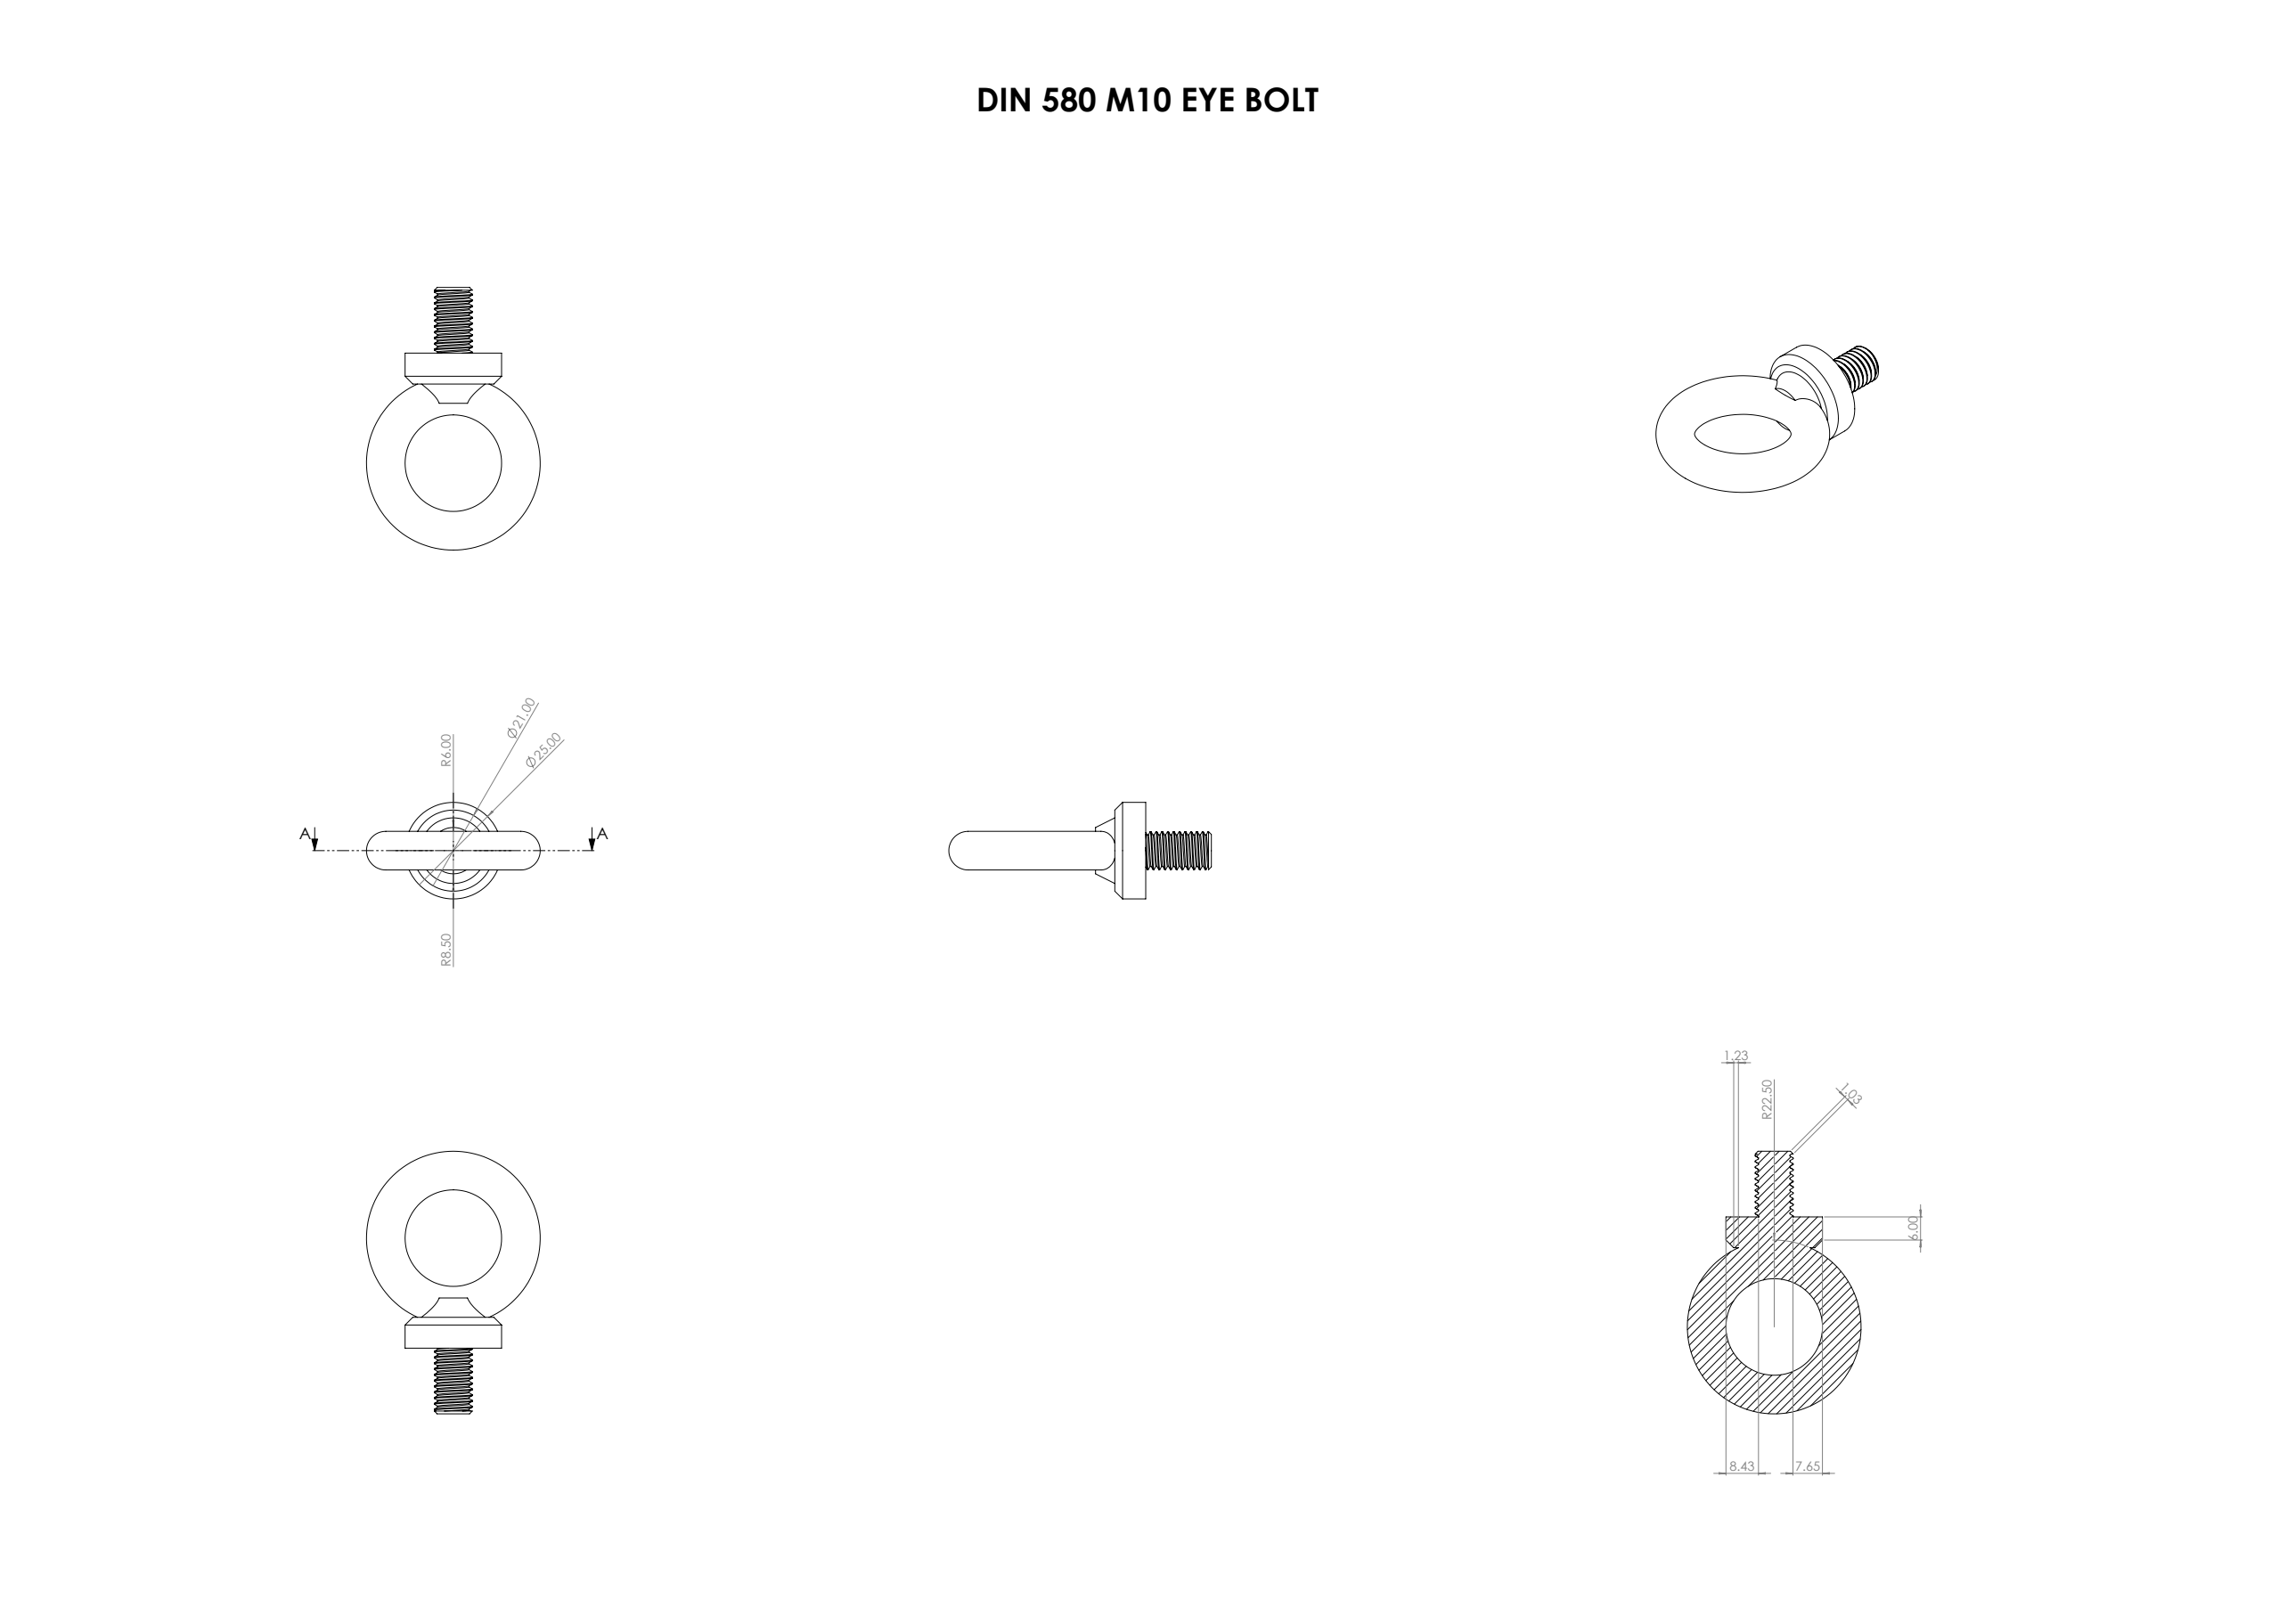
ISO-10303-21;
HEADER;
/* Generated by software containing ST-Developer
 * from STEP Tools, Inc. (www.steptools.com) 
 */

FILE_DESCRIPTION(
/* description */ (''),
/* implementation_level */ '2;1');

FILE_NAME(
/* name */ '15_DIN_580_M10_Eye_Bolt.step',
/* time_stamp */ '2026-10-20T10:03:03-07:00',
/* author */ (''),
/* organization */ (''),
/* preprocessor_version */ 'ST-DEVELOPER v20.2',
/* originating_system */ 'Autodesk Translation Framework v15.15.0.0',
/* authorisation */ '');

FILE_SCHEMA (('AUTOMOTIVE_DESIGN { 1 0 10303 214 3 1 1 }'));
ENDSEC;

DATA;
#10=MECHANICAL_DESIGN_GEOMETRIC_PRESENTATION_REPRESENTATION('',(#537),#71492);
#380=TOROIDAL_SURFACE('',#30209,1.75,0.5);
#394=SHAPE_REPRESENTATION_RELATIONSHIP('SRR','None',#71615,#413);
#413=ADVANCED_BREP_SHAPE_REPRESENTATION('',(#432),#71485);
#432=MANIFOLD_SOLID_BREP('Eye bolt',#28471);
#537=STYLED_ITEM('',(#71894),#432);
#909=B_SPLINE_CURVE_WITH_KNOTS('',3,(#56996,#56997,#56998,#56999,#57000,
#57001,#57002,#57003,#57004,#57005),.UNSPECIFIED.,.F.,.F.,(4,3,3,4),(-4.09323272002469,
-3.95713141738306,-2.9678485630373,-2.06652207565085),.UNSPECIFIED.);
#910=B_SPLINE_CURVE_WITH_KNOTS('',3,(#57008,#57009,#57010,#57011,#57012,
#57013,#57014,#57015,#57016,#57017),.UNSPECIFIED.,.F.,.F.,(4,3,3,4),(0.,
0.494641427172876,0.989282854345763,1.11488200921591),.UNSPECIFIED.);
#911=B_SPLINE_CURVE_WITH_KNOTS('',3,(#57022,#57023,#57024,#57025,#57026,
#57027,#57028,#57029,#57030,#57031,#57032,#57033,#57034,#57035,#57036,#57037,
#57038,#57039,#57040,#57041,#57042,#57043),.UNSPECIFIED.,.F.,.F.,(4,3,3,
3,3,3,3,4),(-10.3764180272043,-9.89282854345765,-8.90354568911189,-7.91426283476612,
-6.92497998042036,-5.93569712607459,-4.94641427172883,-4.09323272002469),
 .UNSPECIFIED.);
#912=B_SPLINE_CURVE_WITH_KNOTS('',3,(#57044,#57045,#57046,#57047,#57048,
#57049,#57050,#57051,#57052,#57053,#57054,#57055,#57056,#57057,#57058,#57059,
#57060,#57061,#57062,#57063,#57064,#57065),.UNSPECIFIED.,.F.,.F.,(4,3,3,
3,3,3,3,4),(1.11488200921591,1.97856570869153,2.9678485630373,3.95713141738306,
4.94641427172883,5.93569712607459,6.92497998042036,7.39806731639549),
 .UNSPECIFIED.);
#913=B_SPLINE_CURVE_WITH_KNOTS('',3,(#57070,#57071,#57072,#57073,#57074,
#57075,#57076,#57077,#57078,#57079,#57080,#57081,#57082,#57083,#57084,#57085,
#57086,#57087,#57088,#57089,#57090,#57091),.UNSPECIFIED.,.F.,.F.,(4,3,3,
3,3,3,3,4),(-16.6596033343839,-15.8285256695322,-14.8392428151865,-13.8499599608407,
-12.860677106495,-11.8713942521492,-10.8821113978034,-10.3764180272043),
 .UNSPECIFIED.);
#914=B_SPLINE_CURVE_WITH_KNOTS('',3,(#57092,#57093,#57094,#57095,#57096,
#57097,#57098,#57099,#57100,#57101,#57102,#57103,#57104,#57105,#57106,#57107,
#57108,#57109,#57110,#57111,#57112,#57113),.UNSPECIFIED.,.F.,.F.,(4,3,3,
3,3,3,3,4),(7.39806731639549,7.91426283476612,8.90354568911189,9.89282854345766,
10.8821113978034,11.8713942521492,12.860677106495,13.6812526235751),
 .UNSPECIFIED.);
#915=B_SPLINE_CURVE_WITH_KNOTS('',3,(#57118,#57119,#57120,#57121,#57122,
#57123,#57124,#57125,#57126,#57127,#57128,#57129,#57130,#57131,#57132,#57133,
#57134,#57135,#57136,#57137,#57138,#57139,#57140,#57141,#57142),
 .UNSPECIFIED.,.F.,.F.,(4,3,3,3,3,3,3,3,4),(-22.9427886415635,-22.7535056499526,
-21.7642227956068,-20.7749399412611,-19.7856570869153,-18.7963742325695,
-17.8070913782238,-16.817808523878,-16.6596033343839),.UNSPECIFIED.);
#916=B_SPLINE_CURVE_WITH_KNOTS('',3,(#57143,#57144,#57145,#57146,#57147,
#57148,#57149,#57150,#57151,#57152,#57153,#57154,#57155,#57156,#57157,#57158,
#57159,#57160,#57161,#57162,#57163,#57164,#57165,#57166,#57167),
 .UNSPECIFIED.,.F.,.F.,(4,3,3,3,3,3,3,3,4),(13.6812526235751,13.8499599608407,
14.8392428151865,15.8285256695323,16.817808523878,17.8070913782238,18.7963742325695,
19.7856570869153,19.9644379307547),.UNSPECIFIED.);
#917=B_SPLINE_CURVE_WITH_KNOTS('',3,(#57172,#57173,#57174,#57175,#57176,
#57177,#57178,#57179,#57180,#57181,#57182,#57183,#57184,#57185,#57186,#57187,
#57188,#57189,#57190,#57191,#57192,#57193),.UNSPECIFIED.,.F.,.F.,(4,3,3,
3,3,3,3,4),(-29.225973948743,-28.6892027760272,-27.6999199216814,-26.7106370673357,
-25.7213542129899,-24.7320713586441,-23.7427885042984,-22.9427886415635),
 .UNSPECIFIED.);
#918=B_SPLINE_CURVE_WITH_KNOTS('',3,(#57194,#57195,#57196,#57197,#57198,
#57199,#57200,#57201,#57202,#57203,#57204,#57205,#57206,#57207,#57208,#57209,
#57210,#57211,#57212,#57213,#57214,#57215),.UNSPECIFIED.,.F.,.F.,(4,3,3,
3,3,3,3,4),(19.9644379307547,20.7749399412611,21.7642227956068,22.7535056499526,
23.7427885042984,24.7320713586441,25.7213542129899,26.2476232379343),
 .UNSPECIFIED.);
#919=B_SPLINE_CURVE_WITH_KNOTS('',3,(#57220,#57221,#57222,#57223,#57224,
#57225,#57226,#57227,#57228,#57229,#57230,#57231,#57232,#57233,#57234,#57235,
#57236,#57237,#57238,#57239,#57240,#57241),.UNSPECIFIED.,.F.,.F.,(4,3,3,
3,3,3,3,4),(-35.5091592559226,-34.6248999021018,-33.635617047756,-32.6463341934103,
-31.6570513390645,-30.6677684847187,-29.678485630373,-29.225973948743),
 .UNSPECIFIED.);
#920=B_SPLINE_CURVE_WITH_KNOTS('',3,(#57242,#57243,#57244,#57245,#57246,
#57247,#57248,#57249,#57250,#57251,#57252,#57253,#57254,#57255,#57256,#57257,
#57258,#57259,#57260,#57261,#57262,#57263),.UNSPECIFIED.,.F.,.F.,(4,3,3,
3,3,3,3,4),(26.2476232379343,26.7106370673357,27.6999199216814,28.6892027760272,
29.678485630373,30.6677684847187,31.6570513390645,32.5308085451138),
 .UNSPECIFIED.);
#921=B_SPLINE_CURVE_WITH_KNOTS('',3,(#57268,#57269,#57270,#57271,#57272,
#57273,#57274,#57275,#57276,#57277,#57278,#57279,#57280,#57281,#57282,#57283,
#57284,#57285,#57286,#57287,#57288,#57289,#57290,#57291,#57292),
 .UNSPECIFIED.,.F.,.F.,(4,3,3,3,3,3,3,3,4),(-41.7923445631022,-41.5498798825222,
-40.5605970281764,-39.5713141738306,-38.5820313194849,-37.5927484651391,
-36.6034656107933,-35.6141827564476,-35.5091592559226),.UNSPECIFIED.);
#922=B_SPLINE_CURVE_WITH_KNOTS('',3,(#57293,#57294,#57295,#57296,#57297,
#57298,#57299,#57300,#57301,#57302,#57303,#57304,#57305,#57306,#57307,#57308,
#57309,#57310,#57311,#57312,#57313,#57314,#57315,#57316,#57317),
 .UNSPECIFIED.,.F.,.F.,(4,3,3,3,3,3,3,3,4),(32.5308085451138,32.6463341934103,
33.635617047756,34.6248999021018,35.6141827564476,36.6034656107933,37.5927484651391,
38.5820313194849,38.8139938522934),.UNSPECIFIED.);
#923=B_SPLINE_CURVE_WITH_KNOTS('',3,(#57322,#57323,#57324,#57325,#57326,
#57327,#57328,#57329,#57330,#57331,#57332,#57333,#57334,#57335,#57336,#57337,
#57338,#57339,#57340,#57341,#57342,#57343),.UNSPECIFIED.,.F.,.F.,(4,3,3,
3,3,3,3,4),(-48.0755298702818,-47.4855770085967,-46.496294154251,-45.5070112999052,
-44.5177284455594,-43.5284455912137,-42.5391627368679,-41.7923445631022),
 .UNSPECIFIED.);
#924=B_SPLINE_CURVE_WITH_KNOTS('',3,(#57344,#57345,#57346,#57347,#57348,
#57349,#57350,#57351,#57352,#57353,#57354,#57355,#57356,#57357,#57358,#57359,
#57360,#57361,#57362,#57363,#57364,#57365),.UNSPECIFIED.,.F.,.F.,(4,3,3,
3,3,3,3,4),(38.8139938522934,39.5713141738306,40.5605970281764,41.5498798825221,
42.5391627368679,43.5284455912137,44.5177284455594,45.097179159473),
 .UNSPECIFIED.);
#925=B_SPLINE_CURVE_WITH_KNOTS('',3,(#57370,#57371,#57372,#57373,#57374,
#57375,#57376,#57377,#57378,#57379,#57380,#57381,#57382,#57383,#57384,#57385,
#57386,#57387,#57388,#57389,#57390,#57391),.UNSPECIFIED.,.F.,.F.,(4,3,3,
3,3,3,3,4),(-54.3587151774614,-53.4212741346713,-52.4319912803256,-51.4427084259798,
-50.453425571634,-49.4641427172883,-48.4748598629425,-48.0755298702818),
 .UNSPECIFIED.);
#926=B_SPLINE_CURVE_WITH_KNOTS('',3,(#57392,#57393,#57394,#57395,#57396,
#57397,#57398,#57399,#57400,#57401,#57402,#57403,#57404,#57405,#57406,#57407,
#57408,#57409,#57410,#57411,#57412,#57413),.UNSPECIFIED.,.F.,.F.,(4,3,3,
3,3,3,3,4),(45.097179159473,45.5070112999052,46.496294154251,47.4855770085967,
48.4748598629425,49.4641427172883,50.4534255716341,51.3803644666526),
 .UNSPECIFIED.);
#927=B_SPLINE_CURVE_WITH_KNOTS('',3,(#57418,#57419,#57420,#57421,#57422,
#57423,#57424,#57425,#57426,#57427,#57428,#57429,#57430,#57431,#57432,#57433,
#57434,#57435,#57436,#57437,#57438,#57439,#57440,#57441,#57442),
 .UNSPECIFIED.,.F.,.F.,(4,3,3,3,3,3,3,3,4),(-60.641900484641,-60.3462541150917,
-59.3569712607459,-58.3676884064002,-57.3784055520544,-56.3891226977086,
-55.3998398433629,-54.4105569890171,-54.3587151774614),.UNSPECIFIED.);
#928=B_SPLINE_CURVE_WITH_KNOTS('',3,(#57443,#57444,#57445,#57446,#57447,
#57448,#57449,#57450,#57451,#57452,#57453,#57454,#57455,#57456,#57457,#57458,
#57459,#57460,#57461,#57462,#57463,#57464,#57465,#57466,#57467),
 .UNSPECIFIED.,.F.,.F.,(4,3,3,3,3,3,3,3,4),(51.3803644666526,51.4427084259798,
52.4319912803256,53.4212741346713,54.4105569890171,55.3998398433629,56.3891226977086,
57.3784055520544,57.6635497738322),.UNSPECIFIED.);
#929=B_SPLINE_CURVE_WITH_KNOTS('',3,(#57472,#57473,#57474,#57475,#57476,
#57477,#57478,#57479,#57480,#57481,#57482,#57483,#57484,#57485,#57486,#57487,
#57488,#57489,#57490,#57491,#57492,#57493),.UNSPECIFIED.,.F.,.F.,(4,3,3,
3,3,3,3,4),(-66.9250857918206,-66.2819512411663,-65.2926683868205,-64.3033855324747,
-63.314102678129,-62.3248198237832,-61.3355369694375,-60.641900484641),
 .UNSPECIFIED.);
#930=B_SPLINE_CURVE_WITH_KNOTS('',3,(#57494,#57495,#57496,#57497,#57498,
#57499,#57500,#57501,#57502,#57503,#57504,#57505,#57506,#57507,#57508,#57509,
#57510,#57511,#57512,#57513,#57514,#57515),.UNSPECIFIED.,.F.,.F.,(4,3,3,
3,3,3,3,4),(57.6635497738322,58.3676884064002,59.3569712607459,60.3462541150917,
61.3355369694375,62.3248198237832,63.314102678129,63.9467350810118),
 .UNSPECIFIED.);
#931=B_SPLINE_CURVE_WITH_KNOTS('',3,(#57521,#57522,#57523,#57524,#57525),
 .UNSPECIFIED.,.F.,.F.,(4,1,4),(78.5398163397448,78.8859646434363,79.7872911308227),
 .UNSPECIFIED.);
#932=B_SPLINE_CURVE_WITH_KNOTS('',3,(#57528,#57529,#57530,#57531),
 .UNSPECIFIED.,.F.,.F.,(4,4),(78.5398163397448,78.5489786101027),
 .UNSPECIFIED.);
#933=B_SPLINE_CURVE_WITH_KNOTS('',3,(#57536,#57537,#57538,#57539,#57540,
#57541,#57542,#57543,#57544,#57545),.UNSPECIFIED.,.F.,.F.,(4,1,1,1,1,1,
1,4),(72.2566310325653,72.9502675173617,73.9395503717074,74.9288332260532,
75.918116080399,76.9073989347447,77.8966817890905,78.5398163397448),
 .UNSPECIFIED.);
#934=B_SPLINE_CURVE_WITH_KNOTS('',3,(#57546,#57547,#57548,#57549,#57550,
#57551,#57552,#57553,#57554,#57555,#57556),.UNSPECIFIED.,.F.,.F.,(4,1,1,
1,1,1,1,1,4),(72.2566310325652,72.6132814840281,73.6025643383739,74.5918471927197,
75.5811300470654,76.5704129014112,77.5596957557569,78.0543371829298,78.5398163397448),
 .UNSPECIFIED.);
#935=B_SPLINE_CURVE_WITH_KNOTS('',3,(#57561,#57562,#57563,#57564,#57565,
#57566,#57567,#57568,#57569,#57570,#57571),.UNSPECIFIED.,.F.,.F.,(4,1,1,
1,1,1,1,1,4),(65.9734457253856,66.0252875369413,67.0145703912871,68.0038532456329,
68.9931360999786,69.9824189543244,70.9717018086701,71.9609846630159,72.2566310325653),
 .UNSPECIFIED.);
#936=B_SPLINE_CURVE_WITH_KNOTS('',3,(#57572,#57573,#57574,#57575,#57576,
#57577,#57578,#57579,#57580,#57581),.UNSPECIFIED.,.F.,.F.,(4,1,1,1,1,1,
1,4),(65.9734457253856,66.6775843579535,67.6668672122993,68.6561500666451,
69.6454329209908,70.6347157753366,71.6239986296824,72.2566310325652),
 .UNSPECIFIED.);
#937=B_SPLINE_CURVE_WITH_KNOTS('',3,(#57586,#57587,#57588,#57589,#57590,
#57591,#57592,#57593,#57594,#57595),.UNSPECIFIED.,.F.,.F.,(4,1,1,1,1,1,
1,4),(59.6902604182061,60.0895904108667,61.0788732652125,62.0681561195583,
63.057438973904,64.0467218282498,65.0360046825956,65.9734457253856),
 .UNSPECIFIED.);
#938=B_SPLINE_CURVE_WITH_KNOTS('',3,(#57596,#57597,#57598,#57599,#57600,
#57601,#57602,#57603,#57604,#57605,#57606),.UNSPECIFIED.,.F.,.F.,(4,1,1,
1,1,1,1,1,4),(59.6902604182061,59.7526043775332,60.7418872318789,61.7311700862247,
62.7204529405705,63.7097357949162,64.699018649262,65.6883015036078,65.9734457253856),
 .UNSPECIFIED.);
#939=B_SPLINE_CURVE_WITH_KNOTS('',3,(#57611,#57612,#57613,#57614,#57615,
#57616,#57617,#57618,#57619,#57620),.UNSPECIFIED.,.F.,.F.,(4,1,1,1,1,1,
1,4),(53.4070751110265,54.1538932847921,55.1431761391379,56.1324589934837,
57.1217418478294,58.1110247021752,59.100307556521,59.6902604182061),
 .UNSPECIFIED.);
#940=B_SPLINE_CURVE_WITH_KNOTS('',3,(#57621,#57622,#57623,#57624,#57625,
#57626,#57627,#57628,#57629,#57630),.UNSPECIFIED.,.F.,.F.,(4,1,1,1,1,1,
1,4),(53.4070751110265,53.8169072514586,54.8061901058043,55.7954729601501,
56.7847558144959,57.7740386688416,58.7633215231874,59.6902604182061),
 .UNSPECIFIED.);
#941=B_SPLINE_CURVE_WITH_KNOTS('',3,(#57635,#57636,#57637,#57638,#57639,
#57640,#57641,#57642,#57643,#57644,#57645),.UNSPECIFIED.,.F.,.F.,(4,1,1,
1,1,1,1,1,4),(47.1238898038469,47.2289133043718,48.2181961587175,49.2074790130633,
50.1967618674091,51.1860447217548,52.1753275761006,53.1646104304464,53.4070751110265),
 .UNSPECIFIED.);
#942=B_SPLINE_CURVE_WITH_KNOTS('',3,(#57646,#57647,#57648,#57649,#57650,
#57651,#57652,#57653,#57654,#57655),.UNSPECIFIED.,.F.,.F.,(4,1,1,1,1,1,
1,4),(47.1238898038469,47.881210125384,48.8704929797298,49.8597758340755,
50.8490586884213,51.8383415427671,52.8276243971128,53.4070751110265),
 .UNSPECIFIED.);
#943=B_SPLINE_CURVE_WITH_KNOTS('',3,(#57660,#57661,#57662,#57663,#57664,
#57665,#57666,#57667,#57668,#57669),.UNSPECIFIED.,.F.,.F.,(4,1,1,1,1,1,
1,4),(40.8407044966673,41.2932161782972,42.2824990326429,43.2717818869887,
44.2610647413345,45.2503475956803,46.239630450026,47.1238898038469),
 .UNSPECIFIED.);
#944=B_SPLINE_CURVE_WITH_KNOTS('',3,(#57670,#57671,#57672,#57673,#57674,
#57675,#57676,#57677,#57678,#57679,#57680),.UNSPECIFIED.,.F.,.F.,(4,1,1,
1,1,1,1,1,4),(40.8407044966673,40.9562301449636,41.9455129993094,42.9347958536552,
43.9240787080009,44.9133615623467,45.9026444166925,46.8919272710382,47.1238898038469),
 .UNSPECIFIED.);
#945=B_SPLINE_CURVE_WITH_KNOTS('',3,(#57685,#57686,#57687,#57688,#57689,
#57690,#57691,#57692,#57693,#57694),.UNSPECIFIED.,.F.,.F.,(4,1,1,1,1,1,
1,4),(34.5575191894877,35.3575190522226,36.3468019065684,37.3360847609141,
38.3253676152599,39.3146504696057,40.3039333239514,40.8407044966673),
 .UNSPECIFIED.);
#946=B_SPLINE_CURVE_WITH_KNOTS('',3,(#57695,#57696,#57697,#57698,#57699,
#57700,#57701,#57702,#57703,#57704),.UNSPECIFIED.,.F.,.F.,(4,1,1,1,1,1,
1,4),(34.5575191894877,35.020533018889,36.0098158732348,36.9990987275806,
37.9883815819263,38.9776644362721,39.9669472906179,40.8407044966673),
 .UNSPECIFIED.);
#947=B_SPLINE_CURVE_WITH_KNOTS('',3,(#57709,#57710,#57711,#57712,#57713,
#57714,#57715,#57716,#57717,#57718,#57719),.UNSPECIFIED.,.F.,.F.,(4,1,1,
1,1,1,1,1,4),(28.2743338823081,28.4325390718022,29.421821926148,30.4111047804938,
31.4003876348395,32.3896704891853,33.3789533435311,34.3682361978768,34.5575191894877),
 .UNSPECIFIED.);
#948=B_SPLINE_CURVE_WITH_KNOTS('',3,(#57720,#57721,#57722,#57723,#57724,
#57725,#57726,#57727,#57728,#57729),.UNSPECIFIED.,.F.,.F.,(4,1,1,1,1,1,
1,4),(28.2743338823081,29.0848358928144,30.0741187471602,31.063401601506,
32.0526844558517,33.0419673101975,34.0312501645433,34.5575191894877),
 .UNSPECIFIED.);
#949=B_SPLINE_CURVE_WITH_KNOTS('',3,(#57734,#57735,#57736,#57737,#57738,
#57739,#57740,#57741,#57742,#57743),.UNSPECIFIED.,.F.,.F.,(4,1,1,1,1,1,
1,4),(21.9911485751285,22.4968419457276,23.4861248000734,24.4754076544192,
25.4646905087649,26.4539733631107,27.4432562174565,28.2743338823081),
 .UNSPECIFIED.);
#950=B_SPLINE_CURVE_WITH_KNOTS('',3,(#57744,#57745,#57746,#57747,#57748,
#57749,#57750,#57751,#57752,#57753,#57754),.UNSPECIFIED.,.F.,.F.,(4,1,1,
1,1,1,1,1,4),(21.9911485751285,22.1598559123941,23.1491387667399,24.1384216210856,
25.1277044754314,26.1169873297771,27.1062701841229,28.0955530384687,28.2743338823081),
 .UNSPECIFIED.);
#951=B_SPLINE_CURVE_WITH_KNOTS('',3,(#57759,#57760,#57761,#57762,#57763,
#57764,#57765,#57766,#57767,#57768),.UNSPECIFIED.,.F.,.F.,(4,1,1,1,1,1,
1,4),(15.7079632679489,16.561144819653,17.5504276739988,18.5397105283446,
19.5289933826903,20.5182762370361,21.5075590913819,21.9911485751285),
 .UNSPECIFIED.);
#952=B_SPLINE_CURVE_WITH_KNOTS('',3,(#57769,#57770,#57771,#57772,#57773,
#57774,#57775,#57776,#57777,#57778),.UNSPECIFIED.,.F.,.F.,(4,1,1,1,1,1,
1,4),(15.7079632679489,16.2241587863195,17.2134416406653,18.202724495011,
19.1920073493568,20.1812902037026,21.1705730580483,21.9911485751285),
 .UNSPECIFIED.);
#953=B_SPLINE_CURVE_WITH_KNOTS('',3,(#57784,#57785,#57786,#57787,#57788,
#57789),.UNSPECIFIED.,.F.,.F.,(4,2,4),(-0.342456092017903,-0.262804961413355,
0.),.UNSPECIFIED.);
#954=B_SPLINE_CURVE_WITH_KNOTS('',3,(#57791,#57792,#57793,#57794,#57795,
#57796,#57797,#57798,#57799,#57800,#57801,#57802),.UNSPECIFIED.,.F.,.F.,
(4,2,2,2,2,4),(0.,0.178010957135692,0.381093675614414,0.596885981784515,
0.750004601526435,0.833159445966906),.UNSPECIFIED.);
#955=B_SPLINE_CURVE_WITH_KNOTS('',3,(#57804,#57805,#57806,#57807,#57808,
#57809,#57810,#57811,#57812,#57813,#57814,#57815,#57816,#57817),
 .UNSPECIFIED.,.F.,.F.,(4,2,2,2,2,2,4),(2.8879030854515,2.90631755511173,
3.01588868292827,3.10104216567944,3.18619564843061,3.29576677624714,3.31418124590738),
 .UNSPECIFIED.);
#956=B_SPLINE_CURVE_WITH_KNOTS('',3,(#57819,#57820,#57821,#57822,#57823,
#57824,#57825,#57826,#57827,#57828,#57829,#57830),.UNSPECIFIED.,.F.,.F.,
(4,2,2,2,2,4),(0.,0.182810359067708,0.452655692105918,0.783610652837132,
0.960006030065839,1.14418486243573),.UNSPECIFIED.);
#957=B_SPLINE_CURVE_WITH_KNOTS('',3,(#57832,#57833,#57834,#57835,#57836,
#57837),.UNSPECIFIED.,.F.,.F.,(4,2,4),(3.5322737051841,3.79507866659746,
3.87472979720201),.UNSPECIFIED.);
#958=B_SPLINE_CURVE_WITH_KNOTS('',3,(#57841,#57842,#57843,#57844,#57845,
#57846),.UNSPECIFIED.,.F.,.F.,(4,2,4),(3.1898176131662,3.26946874377075,
3.5322737051841),.UNSPECIFIED.);
#959=B_SPLINE_CURVE_WITH_KNOTS('',3,(#57848,#57849,#57850,#57851,#57852,
#57853,#57854,#57855,#57856,#57857,#57858,#57859),.UNSPECIFIED.,.F.,.F.,
(4,2,2,2,2,4),(0.,0.178010957135693,0.381093675614418,0.59688598178454,
0.750004601526475,0.833159445966973),.UNSPECIFIED.);
#960=B_SPLINE_CURVE_WITH_KNOTS('',3,(#57861,#57862,#57863,#57864,#57865,
#57866,#57867,#57868,#57869,#57870,#57871,#57872,#57873,#57874),
 .UNSPECIFIED.,.F.,.F.,(4,2,2,2,2,2,4),(0.820541641665208,0.838956111325442,
0.948527239141976,1.03368072189315,1.11883420464432,1.22840533246085,1.24681980212109),
 .UNSPECIFIED.);
#961=B_SPLINE_CURVE_WITH_KNOTS('',3,(#57876,#57877,#57878,#57879,#57880,
#57881,#57882,#57883,#57884,#57885,#57886,#57887),.UNSPECIFIED.,.F.,.F.,
(4,2,2,2,2,4),(0.,0.182810359067185,0.452655692103104,0.783610652831579,
0.960006030058821,1.14418486242717),.UNSPECIFIED.);
#962=B_SPLINE_CURVE_WITH_KNOTS('',3,(#57888,#57889,#57890,#57891,#57892,
#57893),.UNSPECIFIED.,.F.,.F.,(4,2,4),(0.,0.262804961413355,0.342456092017903),
 .UNSPECIFIED.);
#963=B_SPLINE_CURVE_WITH_KNOTS('',3,(#57909,#57910,#57911,#57912,#57913,
#57914,#57915,#57916,#57917,#57918,#57919,#57920,#57921,#57922,#57923,#57924,
#57925,#57926,#57927,#57928,#57929,#57930,#57931,#57932,#57933,#57934,#57935,
#57936,#57937,#57938,#57939,#57940,#57941,#57942,#57943,#57944,#57945,#57946,
#57947,#57948,#57949,#57950,#57951,#57952,#57953,#57954,#57955,#57956,#57957,
#57958,#57959,#57960,#57961,#57962,#57963,#57964,#57965,#57966,#57967,#57968,
#57969,#57970,#57971,#57972,#57973,#57974,#57975),.UNSPECIFIED.,.F.,.F.,
(4,3,3,3,3,3,3,3,3,3,3,3,3,3,3,3,3,3,3,3,3,3,4),(-0.93774096308181,-0.870261948404392,
-0.832251019814623,-0.812039353702878,-0.742348954142412,-0.729339847034109,
-0.705081468871194,-0.634283519265674,-0.572488451018333,-0.549579435213131,
-0.530963570226855,-0.510693382770993,-0.438960472290944,-0.388997500739232,
-0.372134856040166,-0.354858390446,-0.276993114348998,-0.218594157276247,
-0.196204166307054,-0.17703031168743,-0.099567067450566,-0.043397286057993,
0.),.UNSPECIFIED.);
#964=B_SPLINE_CURVE_WITH_KNOTS('',3,(#57977,#57978,#57979,#57980,#57981,
#57982,#57983,#57984,#57985,#57986,#57987,#57988,#57989,#57990,#57991,#57992,
#57993,#57994,#57995,#57996,#57997,#57998,#57999,#58000,#58001,#58002,#58003,
#58004,#58005,#58006,#58007,#58008,#58009,#58010,#58011,#58012,#58013,#58014,
#58015,#58016,#58017,#58018,#58019,#58020,#58021,#58022,#58023,#58024,#58025,
#58026,#58027,#58028,#58029,#58030,#58031,#58032,#58033,#58034,#58035,#58036,
#58037,#58038,#58039,#58040,#58041,#58042,#58043),.UNSPECIFIED.,.F.,.F.,
(4,3,3,3,3,3,3,3,3,3,3,3,3,3,3,3,3,3,3,3,3,3,4),(-0.933975894023158,-0.856824867797122,
-0.821914501343845,-0.791558113020374,-0.71597790947688,-0.694994410329363,
-0.668582197141203,-0.594616471062628,-0.530120471538128,-0.507052841767612,
-0.490181983238915,-0.465624472013627,-0.393047138731511,-0.348092731553511,
-0.32871533726739,-0.312541480427752,-0.242076479471633,-0.190609197809111,
-0.162579557995071,-0.14514061306184,-0.078314656879451,-0.0362073528215457,
0.),.UNSPECIFIED.);
#965=B_SPLINE_CURVE_WITH_KNOTS('',3,(#58356,#58357,#58358,#58359,#58360,
#58361,#58362,#58363,#58364),.UNSPECIFIED.,.F.,.F.,(4,1,1,1,1,1,4),(11.6147305479242,
12.1093719750971,12.60401340227,13.5932962566158,14.5825791109615,15.5718619653073,
15.7079632679489),.UNSPECIFIED.);
#966=B_SPLINE_CURVE_WITH_KNOTS('',3,(#58365,#58366,#58367,#58368,#58369,
#58370,#58371,#58372,#58373,#58374,#58375,#58376,#58377,#58378,#58379,#58380,
#58381,#58382,#58383,#58384,#58385,#58386,#58387,#58388,#58389,#58390,#58391,
#58392,#58393,#58394,#58395,#58396,#58397,#58398,#58399,#58400,#58401,#58402,
#58403,#58404,#58405,#58406,#58407,#58408,#58409,#58410,#58411,#58412,#58413,
#58414,#58415,#58416,#58417,#58418,#58419,#58420,#58421,#58422,#58423,#58424,
#58425,#58426,#58427,#58428,#58429,#58430,#58431),.UNSPECIFIED.,.F.,.F.,
(4,3,3,3,3,3,3,3,3,3,3,3,3,3,3,3,3,3,3,3,3,3,4),(-0.933975894023119,-0.890767895830556,
-0.832649055223636,-0.807165334613026,-0.784870232004528,-0.708420338291616,
-0.684040660118115,-0.663611018024939,-0.589324938941615,-0.542495792243922,
-0.504321658003645,-0.487154884783798,-0.425817170975192,-0.367338377334077,
-0.338840187897342,-0.316929096908672,-0.246728742864094,-0.207915887991521,
-0.16973711093609,-0.149619355722235,-0.0812991141899627,-0.0146711098764389,
0.),.UNSPECIFIED.);
#967=B_SPLINE_CURVE_WITH_KNOTS('',3,(#58432,#58433,#58434,#58435,#58436,
#58437,#58438,#58439,#58440,#58441,#58442,#58443,#58444,#58445,#58446,#58447),
 .UNSPECIFIED.,.F.,.F.,(4,3,3,3,3,4),(-70.2390826585493,-69.7444412313765,
-69.2497998042036,-68.2605169498578,-67.2712340955121,-66.9250857918206),
 .UNSPECIFIED.);
#968=B_SPLINE_CURVE_WITH_KNOTS('',3,(#58450,#58451,#58452,#58453,#58454,
#58455,#58456,#58457,#58458),.UNSPECIFIED.,.F.,.F.,(4,1,1,1,1,1,4),(10.3764180272042,
11.2777445145907,12.2670273689364,13.2563102232822,14.245593077628,15.2348759319737,
15.7079632679489),.UNSPECIFIED.);
#969=B_SPLINE_CURVE_WITH_KNOTS('',3,(#58764,#58765,#58766,#58767,#58768,
#58769,#58770,#58771,#58772,#58773,#58774,#58775,#58776,#58777,#58778,#58779),
 .UNSPECIFIED.,.F.,.F.,(4,3,3,3,3,4),(63.9467350810118,64.3033855324747,
65.2926683868205,66.2819512411663,67.2712340955121,68.1725605828985),
 .UNSPECIFIED.);
#970=B_SPLINE_CURVE_WITH_KNOTS('',3,(#58780,#58781,#58782,#58783,#58784,
#58785,#58786,#58787,#58788,#58789,#58790,#58791,#58792,#58793,#58794,#58795,
#58796,#58797,#58798,#58799,#58800,#58801,#58802,#58803,#58804,#58805,#58806,
#58807,#58808,#58809,#58810,#58811,#58812,#58813,#58814,#58815,#58816,#58817,
#58818,#58819,#58820,#58821,#58822,#58823,#58824,#58825,#58826,#58827,#58828,
#58829,#58830,#58831,#58832,#58833,#58834,#58835,#58836,#58837,#58838,#58839,
#58840,#58841,#58842,#58843),.UNSPECIFIED.,.F.,.F.,(4,3,3,3,3,3,3,3,3,3,
3,3,3,3,3,3,3,3,3,3,3,4),(-0.937740963081774,-0.901429380350922,-0.842615939984195,
-0.815134419970695,-0.763821611298058,-0.734138838750838,-0.715144480290609,
-0.643654231153057,-0.571972635037333,-0.551702893088566,-0.534998195849319,
-0.470725533976372,-0.413107434862205,-0.384514347555702,-0.359013510944126,
-0.284551929400665,-0.240253137519706,-0.200676800014282,-0.176385565585146,
-0.0995853117506865,-0.0229257113100043,0.),.UNSPECIFIED.);
#1462=B_SPLINE_SURFACE_WITH_KNOTS('',3,3,((#58051,#58052,#58053,#58054,
#58055,#58056,#58057,#58058,#58059,#58060,#58061,#58062,#58063,#58064,#58065,
#58066,#58067,#58068,#58069,#58070,#58071,#58072,#58073,#58074,#58075,#58076,
#58077,#58078,#58079,#58080,#58081,#58082,#58083,#58084,#58085,#58086,#58087,
#58088,#58089,#58090,#58091,#58092,#58093,#58094,#58095,#58096,#58097,#58098,
#58099,#58100,#58101,#58102,#58103,#58104,#58105,#58106,#58107,#58108,#58109,
#58110,#58111,#58112,#58113,#58114,#58115,#58116,#58117,#58118,#58119,#58120,
#58121,#58122,#58123,#58124,#58125,#58126),(#58127,#58128,#58129,#58130,
#58131,#58132,#58133,#58134,#58135,#58136,#58137,#58138,#58139,#58140,#58141,
#58142,#58143,#58144,#58145,#58146,#58147,#58148,#58149,#58150,#58151,#58152,
#58153,#58154,#58155,#58156,#58157,#58158,#58159,#58160,#58161,#58162,#58163,
#58164,#58165,#58166,#58167,#58168,#58169,#58170,#58171,#58172,#58173,#58174,
#58175,#58176,#58177,#58178,#58179,#58180,#58181,#58182,#58183,#58184,#58185,
#58186,#58187,#58188,#58189,#58190,#58191,#58192,#58193,#58194,#58195,#58196,
#58197,#58198,#58199,#58200,#58201,#58202),(#58203,#58204,#58205,#58206,
#58207,#58208,#58209,#58210,#58211,#58212,#58213,#58214,#58215,#58216,#58217,
#58218,#58219,#58220,#58221,#58222,#58223,#58224,#58225,#58226,#58227,#58228,
#58229,#58230,#58231,#58232,#58233,#58234,#58235,#58236,#58237,#58238,#58239,
#58240,#58241,#58242,#58243,#58244,#58245,#58246,#58247,#58248,#58249,#58250,
#58251,#58252,#58253,#58254,#58255,#58256,#58257,#58258,#58259,#58260,#58261,
#58262,#58263,#58264,#58265,#58266,#58267,#58268,#58269,#58270,#58271,#58272,
#58273,#58274,#58275,#58276,#58277,#58278),(#58279,#58280,#58281,#58282,
#58283,#58284,#58285,#58286,#58287,#58288,#58289,#58290,#58291,#58292,#58293,
#58294,#58295,#58296,#58297,#58298,#58299,#58300,#58301,#58302,#58303,#58304,
#58305,#58306,#58307,#58308,#58309,#58310,#58311,#58312,#58313,#58314,#58315,
#58316,#58317,#58318,#58319,#58320,#58321,#58322,#58323,#58324,#58325,#58326,
#58327,#58328,#58329,#58330,#58331,#58332,#58333,#58334,#58335,#58336,#58337,
#58338,#58339,#58340,#58341,#58342,#58343,#58344,#58345,#58346,#58347,#58348,
#58349,#58350,#58351,#58352,#58353,#58354)),.UNSPECIFIED.,.F.,.F.,.F.,(4,
4),(4,1,1,1,1,1,1,1,1,1,1,1,1,1,1,1,1,1,1,1,1,1,1,1,1,1,1,1,1,1,1,1,1,1,
1,1,1,1,1,1,1,1,1,1,1,1,1,1,1,1,1,1,1,1,1,1,1,1,1,1,1,1,1,1,1,1,1,1,1,1,
1,1,1,4),(0.,0.0986691610045069),(11.6147305479242,12.1093719750971,12.60401340227,
13.5932962566158,14.5825791109615,15.5718619653073,16.561144819653,17.5504276739988,
18.5397105283446,19.5289933826903,20.5182762370361,21.5075590913819,22.4968419457276,
23.4861248000734,24.4754076544192,25.4646905087649,26.4539733631107,27.4432562174565,
28.4325390718022,29.421821926148,30.4111047804938,31.4003876348395,32.3896704891853,
33.3789533435311,34.3682361978768,35.3575190522226,36.3468019065684,37.3360847609141,
38.3253676152599,39.3146504696057,40.3039333239514,41.2932161782972,42.2824990326429,
43.2717818869887,44.2610647413345,45.2503475956803,46.239630450026,47.2289133043718,
48.2181961587175,49.2074790130633,50.1967618674091,51.1860447217548,52.1753275761006,
53.1646104304464,54.1538932847921,55.1431761391379,56.1324589934837,57.1217418478294,
58.1110247021752,59.100307556521,60.0895904108667,61.0788732652125,62.0681561195583,
63.057438973904,64.0467218282498,65.0360046825956,66.0252875369413,67.0145703912871,
68.0038532456329,68.9931360999786,69.9824189543244,70.9717018086701,71.9609846630159,
72.9502675173617,73.9395503717074,74.9288332260532,75.918116080399,76.9073989347447,
77.8966817890905,78.8859646434363,79.875247497782,80.8645303521278,81.3591717793007,
81.8538132064736),.UNSPECIFIED.);
#1463=B_SPLINE_SURFACE_WITH_KNOTS('',3,3,((#58460,#58461,#58462,#58463,
#58464,#58465,#58466,#58467,#58468,#58469,#58470,#58471,#58472,#58473,#58474,
#58475,#58476,#58477,#58478,#58479,#58480,#58481,#58482,#58483,#58484,#58485,
#58486,#58487,#58488,#58489,#58490,#58491,#58492,#58493,#58494,#58495,#58496,
#58497,#58498,#58499,#58500,#58501,#58502,#58503,#58504,#58505,#58506,#58507,
#58508,#58509,#58510,#58511,#58512,#58513,#58514,#58515,#58516,#58517,#58518,
#58519,#58520,#58521,#58522,#58523,#58524,#58525,#58526,#58527,#58528,#58529,
#58530,#58531,#58532,#58533,#58534,#58535),(#58536,#58537,#58538,#58539,
#58540,#58541,#58542,#58543,#58544,#58545,#58546,#58547,#58548,#58549,#58550,
#58551,#58552,#58553,#58554,#58555,#58556,#58557,#58558,#58559,#58560,#58561,
#58562,#58563,#58564,#58565,#58566,#58567,#58568,#58569,#58570,#58571,#58572,
#58573,#58574,#58575,#58576,#58577,#58578,#58579,#58580,#58581,#58582,#58583,
#58584,#58585,#58586,#58587,#58588,#58589,#58590,#58591,#58592,#58593,#58594,
#58595,#58596,#58597,#58598,#58599,#58600,#58601,#58602,#58603,#58604,#58605,
#58606,#58607,#58608,#58609,#58610,#58611),(#58612,#58613,#58614,#58615,
#58616,#58617,#58618,#58619,#58620,#58621,#58622,#58623,#58624,#58625,#58626,
#58627,#58628,#58629,#58630,#58631,#58632,#58633,#58634,#58635,#58636,#58637,
#58638,#58639,#58640,#58641,#58642,#58643,#58644,#58645,#58646,#58647,#58648,
#58649,#58650,#58651,#58652,#58653,#58654,#58655,#58656,#58657,#58658,#58659,
#58660,#58661,#58662,#58663,#58664,#58665,#58666,#58667,#58668,#58669,#58670,
#58671,#58672,#58673,#58674,#58675,#58676,#58677,#58678,#58679,#58680,#58681,
#58682,#58683,#58684,#58685,#58686,#58687),(#58688,#58689,#58690,#58691,
#58692,#58693,#58694,#58695,#58696,#58697,#58698,#58699,#58700,#58701,#58702,
#58703,#58704,#58705,#58706,#58707,#58708,#58709,#58710,#58711,#58712,#58713,
#58714,#58715,#58716,#58717,#58718,#58719,#58720,#58721,#58722,#58723,#58724,
#58725,#58726,#58727,#58728,#58729,#58730,#58731,#58732,#58733,#58734,#58735,
#58736,#58737,#58738,#58739,#58740,#58741,#58742,#58743,#58744,#58745,#58746,
#58747,#58748,#58749,#58750,#58751,#58752,#58753,#58754,#58755,#58756,#58757,
#58758,#58759,#58760,#58761,#58762,#58763)),.UNSPECIFIED.,.F.,.F.,.F.,(4,
4),(4,1,1,1,1,1,1,1,1,1,1,1,1,1,1,1,1,1,1,1,1,1,1,1,1,1,1,1,1,1,1,1,1,1,
1,1,1,1,1,1,1,1,1,1,1,1,1,1,1,1,1,1,1,1,1,1,1,1,1,1,1,1,1,1,1,1,1,1,1,1,
1,1,1,4),(0.,0.0986691610045069),(8.30989595155337,8.80453737872625,9.29917880589914,
10.2884616602449,11.2777445145907,12.2670273689364,13.2563102232822,14.245593077628,
15.2348759319737,16.2241587863195,17.2134416406653,18.202724495011,19.1920073493568,
20.1812902037026,21.1705730580483,22.1598559123941,23.1491387667399,24.1384216210856,
25.1277044754314,26.1169873297771,27.1062701841229,28.0955530384687,29.0848358928144,
30.0741187471602,31.063401601506,32.0526844558517,33.0419673101975,34.0312501645433,
35.020533018889,36.0098158732348,36.9990987275806,37.9883815819263,38.9776644362721,
39.9669472906179,40.9562301449636,41.9455129993094,42.9347958536552,43.9240787080009,
44.9133615623467,45.9026444166925,46.8919272710382,47.881210125384,48.8704929797298,
49.8597758340755,50.8490586884213,51.8383415427671,52.8276243971128,53.8169072514586,
54.8061901058043,55.7954729601501,56.7847558144959,57.7740386688416,58.7633215231874,
59.7526043775332,60.7418872318789,61.7311700862247,62.7204529405705,63.7097357949162,
64.699018649262,65.6883015036078,66.6775843579535,67.6668672122993,68.6561500666451,
69.6454329209908,70.6347157753366,71.6239986296824,72.6132814840281,73.6025643383739,
74.5918471927197,75.5811300470654,76.5704129014112,77.5596957557569,78.0543371829298,
78.5489786101027),.UNSPECIFIED.);
#1684=CYLINDRICAL_SURFACE('',#30185,0.4925);
#1685=CYLINDRICAL_SURFACE('',#30187,0.4925);
#1686=CYLINDRICAL_SURFACE('',#30188,0.4925);
#1687=CYLINDRICAL_SURFACE('',#30189,0.4925);
#1688=CYLINDRICAL_SURFACE('',#30190,0.4925);
#1689=CYLINDRICAL_SURFACE('',#30191,0.4925);
#1690=CYLINDRICAL_SURFACE('',#30192,0.4925);
#1691=CYLINDRICAL_SURFACE('',#30193,0.4925);
#1692=CYLINDRICAL_SURFACE('',#30194,0.4925);
#1693=CYLINDRICAL_SURFACE('',#30195,0.4925);
#1694=CYLINDRICAL_SURFACE('',#30196,0.4925);
#1695=CYLINDRICAL_SURFACE('',#30197,0.40705);
#1696=CYLINDRICAL_SURFACE('',#30199,0.40705);
#1697=CYLINDRICAL_SURFACE('',#30200,0.40705);
#1698=CYLINDRICAL_SURFACE('',#30201,0.40705);
#1699=CYLINDRICAL_SURFACE('',#30202,0.40705);
#1700=CYLINDRICAL_SURFACE('',#30203,0.40705);
#1701=CYLINDRICAL_SURFACE('',#30204,0.40705);
#1702=CYLINDRICAL_SURFACE('',#30205,0.40705);
#1703=CYLINDRICAL_SURFACE('',#30206,0.40705);
#1704=CYLINDRICAL_SURFACE('',#30207,0.40705);
#1705=CYLINDRICAL_SURFACE('',#30208,0.40705);
#1706=CYLINDRICAL_SURFACE('',#30226,1.25);
#1707=CYLINDRICAL_SURFACE('',#30229,0.40705);
#1708=CYLINDRICAL_SURFACE('',#30237,0.4925);
#1974=FACE_BOUND('',#5784,.T.);
#1975=FACE_BOUND('',#5790,.T.);
#2533=CIRCLE('',#30186,0.4925);
#2534=CIRCLE('',#30198,0.40705);
#2535=CIRCLE('',#30210,0.5);
#2536=CIRCLE('',#30211,0.5);
#2537=CIRCLE('',#30212,1.25);
#2538=CIRCLE('',#30214,1.05);
#2539=CIRCLE('',#30215,0.85);
#2540=CIRCLE('',#30216,0.85);
#2541=CIRCLE('',#30218,0.6);
#2542=CIRCLE('',#30221,0.6);
#2543=CIRCLE('',#30224,1.25);
#2544=CIRCLE('',#30225,0.4925);
#2545=CIRCLE('',#30227,1.25);
#2546=CIRCLE('',#30230,0.40705);
#2547=CIRCLE('',#30232,0.4925);
#2548=CIRCLE('',#30233,0.4925);
#2549=CIRCLE('',#30235,0.42);
#2889=CONICAL_SURFACE('',#30219,0.75,0.463647609000806);
#2890=CONICAL_SURFACE('',#30220,0.75,0.463647609000806);
#2891=CONICAL_SURFACE('',#30228,1.15,0.785398163397448);
#2892=CONICAL_SURFACE('',#30236,0.46,0.785398163397448);
#4080=FACE_OUTER_BOUND('',#5760,.T.);
#4081=FACE_OUTER_BOUND('',#5761,.T.);
#4082=FACE_OUTER_BOUND('',#5762,.T.);
#4083=FACE_OUTER_BOUND('',#5763,.T.);
#4084=FACE_OUTER_BOUND('',#5764,.T.);
#4085=FACE_OUTER_BOUND('',#5765,.T.);
#4086=FACE_OUTER_BOUND('',#5766,.T.);
#4087=FACE_OUTER_BOUND('',#5767,.T.);
#4088=FACE_OUTER_BOUND('',#5768,.T.);
#4089=FACE_OUTER_BOUND('',#5769,.T.);
#4090=FACE_OUTER_BOUND('',#5770,.T.);
#4091=FACE_OUTER_BOUND('',#5771,.T.);
#4092=FACE_OUTER_BOUND('',#5772,.T.);
#4093=FACE_OUTER_BOUND('',#5773,.T.);
#4094=FACE_OUTER_BOUND('',#5774,.T.);
#4095=FACE_OUTER_BOUND('',#5775,.T.);
#4096=FACE_OUTER_BOUND('',#5776,.T.);
#4097=FACE_OUTER_BOUND('',#5777,.T.);
#4098=FACE_OUTER_BOUND('',#5778,.T.);
#4099=FACE_OUTER_BOUND('',#5779,.T.);
#4100=FACE_OUTER_BOUND('',#5780,.T.);
#4101=FACE_OUTER_BOUND('',#5781,.T.);
#4102=FACE_OUTER_BOUND('',#5782,.T.);
#4103=FACE_OUTER_BOUND('',#5783,.T.);
#4104=FACE_OUTER_BOUND('',#5785,.T.);
#4105=FACE_OUTER_BOUND('',#5786,.T.);
#4106=FACE_OUTER_BOUND('',#5787,.T.);
#4107=FACE_OUTER_BOUND('',#5788,.T.);
#4108=FACE_OUTER_BOUND('',#5789,.T.);
#4109=FACE_OUTER_BOUND('',#5791,.T.);
#4110=FACE_OUTER_BOUND('',#5792,.T.);
#4111=FACE_OUTER_BOUND('',#5793,.T.);
#4112=FACE_OUTER_BOUND('',#5794,.T.);
#4113=FACE_OUTER_BOUND('',#5795,.T.);
#4114=FACE_OUTER_BOUND('',#5796,.T.);
#4115=FACE_OUTER_BOUND('',#5797,.T.);
#4116=FACE_OUTER_BOUND('',#5798,.T.);
#4117=FACE_OUTER_BOUND('',#5799,.T.);
#5760=EDGE_LOOP('',(#23661,#23662,#23663,#23664));
#5761=EDGE_LOOP('',(#23665,#23666,#23667,#23668));
#5762=EDGE_LOOP('',(#23669,#23670,#23671,#23672));
#5763=EDGE_LOOP('',(#23673,#23674,#23675,#23676));
#5764=EDGE_LOOP('',(#23677,#23678,#23679,#23680));
#5765=EDGE_LOOP('',(#23681,#23682,#23683,#23684));
#5766=EDGE_LOOP('',(#23685,#23686,#23687,#23688));
#5767=EDGE_LOOP('',(#23689,#23690,#23691,#23692));
#5768=EDGE_LOOP('',(#23693,#23694,#23695,#23696));
#5769=EDGE_LOOP('',(#23697,#23698,#23699,#23700));
#5770=EDGE_LOOP('',(#23701,#23702,#23703,#23704));
#5771=EDGE_LOOP('',(#23705,#23706,#23707,#23708));
#5772=EDGE_LOOP('',(#23709,#23710,#23711,#23712));
#5773=EDGE_LOOP('',(#23713,#23714,#23715,#23716));
#5774=EDGE_LOOP('',(#23717,#23718,#23719,#23720));
#5775=EDGE_LOOP('',(#23721,#23722,#23723,#23724));
#5776=EDGE_LOOP('',(#23725,#23726,#23727,#23728));
#5777=EDGE_LOOP('',(#23729,#23730,#23731,#23732));
#5778=EDGE_LOOP('',(#23733,#23734,#23735,#23736));
#5779=EDGE_LOOP('',(#23737,#23738,#23739,#23740));
#5780=EDGE_LOOP('',(#23741,#23742,#23743,#23744));
#5781=EDGE_LOOP('',(#23745,#23746,#23747,#23748));
#5782=EDGE_LOOP('',(#23749,#23750,#23751,#23752,#23753,#23754,#23755,#23756,
#23757,#23758,#23759,#23760,#23761,#23762,#23763,#23764));
#5783=EDGE_LOOP('',(#23765));
#5784=EDGE_LOOP('',(#23766,#23767,#23768,#23769));
#5785=EDGE_LOOP('',(#23770,#23771,#23772));
#5786=EDGE_LOOP('',(#23773,#23774,#23775,#23776));
#5787=EDGE_LOOP('',(#23777,#23778,#23779,#23780));
#5788=EDGE_LOOP('',(#23781,#23782,#23783));
#5789=EDGE_LOOP('',(#23784));
#5790=EDGE_LOOP('',(#23785,#23786,#23787,#23788));
#5791=EDGE_LOOP('',(#23789,#23790,#23791,#23792));
#5792=EDGE_LOOP('',(#23793,#23794,#23795,#23796));
#5793=EDGE_LOOP('',(#23797,#23798,#23799,#23800,#23801,#23802,#23803,#23804,
#23805,#23806,#23807,#23808,#23809,#23810,#23811,#23812,#23813,#23814,#23815,
#23816,#23817,#23818,#23819,#23820,#23821,#23822));
#5794=EDGE_LOOP('',(#23823,#23824,#23825,#23826));
#5795=EDGE_LOOP('',(#23827,#23828,#23829,#23830,#23831,#23832,#23833,#23834,
#23835,#23836,#23837,#23838,#23839,#23840,#23841,#23842,#23843,#23844,#23845,
#23846,#23847,#23848,#23849,#23850,#23851,#23852));
#5796=EDGE_LOOP('',(#23853,#23854,#23855,#23856,#23857));
#5797=EDGE_LOOP('',(#23858));
#5798=EDGE_LOOP('',(#23859,#23860,#23861,#23862,#23863,#23864));
#5799=EDGE_LOOP('',(#23865,#23866,#23867,#23868));
#8243=LINE('',#56994,#10731);
#8244=LINE('',#57021,#10732);
#8245=LINE('',#57069,#10733);
#8246=LINE('',#57117,#10734);
#8247=LINE('',#57171,#10735);
#8248=LINE('',#57219,#10736);
#8249=LINE('',#57267,#10737);
#8250=LINE('',#57321,#10738);
#8251=LINE('',#57369,#10739);
#8252=LINE('',#57417,#10740);
#8253=LINE('',#57471,#10741);
#8254=LINE('',#57519,#10742);
#8255=LINE('',#57535,#10743);
#8256=LINE('',#57560,#10744);
#8257=LINE('',#57585,#10745);
#8258=LINE('',#57610,#10746);
#8259=LINE('',#57634,#10747);
#8260=LINE('',#57659,#10748);
#8261=LINE('',#57684,#10749);
#8262=LINE('',#57708,#10750);
#8263=LINE('',#57733,#10751);
#8264=LINE('',#57758,#10752);
#8265=LINE('',#58048,#10753);
#8266=LINE('',#58050,#10754);
#8267=LINE('',#58852,#10755);
#10731=VECTOR('',#35792,0.5);
#10732=VECTOR('',#35797,0.5);
#10733=VECTOR('',#35800,0.5);
#10734=VECTOR('',#35803,0.5);
#10735=VECTOR('',#35806,0.5);
#10736=VECTOR('',#35809,0.5);
#10737=VECTOR('',#35812,0.5);
#10738=VECTOR('',#35815,0.5);
#10739=VECTOR('',#35818,0.5);
#10740=VECTOR('',#35821,0.5);
#10741=VECTOR('',#35824,0.5);
#10742=VECTOR('',#35827,0.40705);
#10743=VECTOR('',#35832,0.40705);
#10744=VECTOR('',#35835,0.40705);
#10745=VECTOR('',#35838,0.40705);
#10746=VECTOR('',#35841,0.40705);
#10747=VECTOR('',#35844,0.40705);
#10748=VECTOR('',#35847,0.40705);
#10749=VECTOR('',#35850,0.40705);
#10750=VECTOR('',#35853,0.40705);
#10751=VECTOR('',#35856,0.40705);
#10752=VECTOR('',#35859,0.40705);
#10753=VECTOR('',#35898,1.25);
#10754=VECTOR('',#35901,1.15);
#10755=VECTOR('',#35918,0.46);
#13078=VERTEX_POINT('',#56992);
#13079=VERTEX_POINT('',#56993);
#13080=VERTEX_POINT('',#56995);
#13081=VERTEX_POINT('',#57006);
#13082=VERTEX_POINT('',#57019);
#13083=VERTEX_POINT('',#57020);
#13084=VERTEX_POINT('',#57067);
#13085=VERTEX_POINT('',#57068);
#13086=VERTEX_POINT('',#57115);
#13087=VERTEX_POINT('',#57116);
#13088=VERTEX_POINT('',#57169);
#13089=VERTEX_POINT('',#57170);
#13090=VERTEX_POINT('',#57217);
#13091=VERTEX_POINT('',#57218);
#13092=VERTEX_POINT('',#57265);
#13093=VERTEX_POINT('',#57266);
#13094=VERTEX_POINT('',#57319);
#13095=VERTEX_POINT('',#57320);
#13096=VERTEX_POINT('',#57367);
#13097=VERTEX_POINT('',#57368);
#13098=VERTEX_POINT('',#57415);
#13099=VERTEX_POINT('',#57416);
#13100=VERTEX_POINT('',#57469);
#13101=VERTEX_POINT('',#57470);
#13102=VERTEX_POINT('',#57517);
#13103=VERTEX_POINT('',#57518);
#13104=VERTEX_POINT('',#57520);
#13105=VERTEX_POINT('',#57526);
#13106=VERTEX_POINT('',#57533);
#13107=VERTEX_POINT('',#57534);
#13108=VERTEX_POINT('',#57558);
#13109=VERTEX_POINT('',#57559);
#13110=VERTEX_POINT('',#57583);
#13111=VERTEX_POINT('',#57584);
#13112=VERTEX_POINT('',#57608);
#13113=VERTEX_POINT('',#57609);
#13114=VERTEX_POINT('',#57632);
#13115=VERTEX_POINT('',#57633);
#13116=VERTEX_POINT('',#57657);
#13117=VERTEX_POINT('',#57658);
#13118=VERTEX_POINT('',#57682);
#13119=VERTEX_POINT('',#57683);
#13120=VERTEX_POINT('',#57706);
#13121=VERTEX_POINT('',#57707);
#13122=VERTEX_POINT('',#57731);
#13123=VERTEX_POINT('',#57732);
#13124=VERTEX_POINT('',#57756);
#13125=VERTEX_POINT('',#57757);
#13126=VERTEX_POINT('',#57780);
#13127=VERTEX_POINT('',#57781);
#13128=VERTEX_POINT('',#57783);
#13129=VERTEX_POINT('',#57790);
#13130=VERTEX_POINT('',#57803);
#13131=VERTEX_POINT('',#57818);
#13132=VERTEX_POINT('',#57831);
#13133=VERTEX_POINT('',#57840);
#13134=VERTEX_POINT('',#57847);
#13135=VERTEX_POINT('',#57860);
#13136=VERTEX_POINT('',#57875);
#13137=VERTEX_POINT('',#57895);
#13138=VERTEX_POINT('',#57906);
#13139=VERTEX_POINT('',#57908);
#13140=VERTEX_POINT('',#57976);
#13141=VERTEX_POINT('',#58046);
#13142=VERTEX_POINT('',#58355);
#13143=VERTEX_POINT('',#58449);
#13144=VERTEX_POINT('',#58845);
#13145=VERTEX_POINT('',#58849);
#16714=EDGE_CURVE('',#13078,#13079,#8243,.T.);
#16715=EDGE_CURVE('',#13078,#13080,#909,.T.);
#16716=EDGE_CURVE('',#13080,#13081,#2533,.T.);
#16717=EDGE_CURVE('',#13081,#13079,#910,.T.);
#16718=EDGE_CURVE('',#13082,#13083,#8244,.T.);
#16719=EDGE_CURVE('',#13082,#13078,#911,.T.);
#16720=EDGE_CURVE('',#13079,#13083,#912,.T.);
#16721=EDGE_CURVE('',#13084,#13085,#8245,.T.);
#16722=EDGE_CURVE('',#13084,#13082,#913,.T.);
#16723=EDGE_CURVE('',#13083,#13085,#914,.T.);
#16724=EDGE_CURVE('',#13086,#13087,#8246,.T.);
#16725=EDGE_CURVE('',#13086,#13084,#915,.T.);
#16726=EDGE_CURVE('',#13085,#13087,#916,.T.);
#16727=EDGE_CURVE('',#13088,#13089,#8247,.T.);
#16728=EDGE_CURVE('',#13088,#13086,#917,.T.);
#16729=EDGE_CURVE('',#13087,#13089,#918,.T.);
#16730=EDGE_CURVE('',#13090,#13091,#8248,.T.);
#16731=EDGE_CURVE('',#13090,#13088,#919,.T.);
#16732=EDGE_CURVE('',#13089,#13091,#920,.T.);
#16733=EDGE_CURVE('',#13092,#13093,#8249,.T.);
#16734=EDGE_CURVE('',#13092,#13090,#921,.T.);
#16735=EDGE_CURVE('',#13091,#13093,#922,.T.);
#16736=EDGE_CURVE('',#13094,#13095,#8250,.T.);
#16737=EDGE_CURVE('',#13094,#13092,#923,.T.);
#16738=EDGE_CURVE('',#13093,#13095,#924,.T.);
#16739=EDGE_CURVE('',#13096,#13097,#8251,.T.);
#16740=EDGE_CURVE('',#13096,#13094,#925,.T.);
#16741=EDGE_CURVE('',#13095,#13097,#926,.T.);
#16742=EDGE_CURVE('',#13098,#13099,#8252,.T.);
#16743=EDGE_CURVE('',#13098,#13096,#927,.T.);
#16744=EDGE_CURVE('',#13097,#13099,#928,.T.);
#16745=EDGE_CURVE('',#13100,#13101,#8253,.T.);
#16746=EDGE_CURVE('',#13100,#13098,#929,.T.);
#16747=EDGE_CURVE('',#13099,#13101,#930,.T.);
#16748=EDGE_CURVE('',#13102,#13103,#8254,.T.);
#16749=EDGE_CURVE('',#13102,#13104,#931,.T.);
#16750=EDGE_CURVE('',#13104,#13105,#2534,.T.);
#16751=EDGE_CURVE('',#13103,#13105,#932,.T.);
#16752=EDGE_CURVE('',#13106,#13107,#8255,.T.);
#16753=EDGE_CURVE('',#13106,#13102,#933,.T.);
#16754=EDGE_CURVE('',#13107,#13103,#934,.T.);
#16755=EDGE_CURVE('',#13108,#13109,#8256,.T.);
#16756=EDGE_CURVE('',#13108,#13106,#935,.T.);
#16757=EDGE_CURVE('',#13109,#13107,#936,.T.);
#16758=EDGE_CURVE('',#13110,#13111,#8257,.T.);
#16759=EDGE_CURVE('',#13110,#13108,#937,.T.);
#16760=EDGE_CURVE('',#13111,#13109,#938,.T.);
#16761=EDGE_CURVE('',#13112,#13113,#8258,.T.);
#16762=EDGE_CURVE('',#13112,#13110,#939,.T.);
#16763=EDGE_CURVE('',#13113,#13111,#940,.T.);
#16764=EDGE_CURVE('',#13114,#13115,#8259,.T.);
#16765=EDGE_CURVE('',#13114,#13112,#941,.T.);
#16766=EDGE_CURVE('',#13115,#13113,#942,.T.);
#16767=EDGE_CURVE('',#13116,#13117,#8260,.T.);
#16768=EDGE_CURVE('',#13116,#13114,#943,.T.);
#16769=EDGE_CURVE('',#13117,#13115,#944,.T.);
#16770=EDGE_CURVE('',#13118,#13119,#8261,.T.);
#16771=EDGE_CURVE('',#13118,#13116,#945,.T.);
#16772=EDGE_CURVE('',#13119,#13117,#946,.T.);
#16773=EDGE_CURVE('',#13120,#13121,#8262,.T.);
#16774=EDGE_CURVE('',#13120,#13118,#947,.T.);
#16775=EDGE_CURVE('',#13121,#13119,#948,.T.);
#16776=EDGE_CURVE('',#13122,#13123,#8263,.T.);
#16777=EDGE_CURVE('',#13122,#13120,#949,.T.);
#16778=EDGE_CURVE('',#13123,#13121,#950,.T.);
#16779=EDGE_CURVE('',#13124,#13125,#8264,.T.);
#16780=EDGE_CURVE('',#13124,#13122,#951,.T.);
#16781=EDGE_CURVE('',#13125,#13123,#952,.T.);
#16782=EDGE_CURVE('',#13126,#13127,#2535,.T.);
#16783=EDGE_CURVE('',#13128,#13126,#953,.T.);
#16784=EDGE_CURVE('',#13129,#13128,#954,.T.);
#16785=EDGE_CURVE('',#13130,#13129,#955,.T.);
#16786=EDGE_CURVE('',#13131,#13130,#956,.T.);
#16787=EDGE_CURVE('',#13132,#13131,#957,.T.);
#16788=EDGE_CURVE('',#13127,#13132,#2536,.T.);
#16789=EDGE_CURVE('',#13127,#13127,#2537,.T.);
#16790=EDGE_CURVE('',#13133,#13132,#958,.T.);
#16791=EDGE_CURVE('',#13134,#13133,#959,.T.);
#16792=EDGE_CURVE('',#13135,#13134,#960,.T.);
#16793=EDGE_CURVE('',#13136,#13135,#961,.T.);
#16794=EDGE_CURVE('',#13126,#13136,#962,.T.);
#16795=EDGE_CURVE('',#13137,#13137,#2538,.T.);
#16796=EDGE_CURVE('',#13129,#13135,#2539,.T.);
#16797=EDGE_CURVE('',#13134,#13130,#2540,.T.);
#16798=EDGE_CURVE('',#13136,#13128,#2541,.T.);
#16799=EDGE_CURVE('',#13131,#13133,#2542,.T.);
#16800=EDGE_CURVE('',#13138,#13138,#2543,.T.);
#16801=EDGE_CURVE('',#13105,#13139,#963,.T.);
#16802=EDGE_CURVE('',#13140,#13104,#964,.T.);
#16803=EDGE_CURVE('',#13139,#13140,#2544,.T.);
#16804=EDGE_CURVE('',#13141,#13141,#2545,.T.);
#16805=EDGE_CURVE('',#13141,#13138,#8265,.T.);
#16806=EDGE_CURVE('',#13137,#13141,#8266,.T.);
#16807=EDGE_CURVE('',#13142,#13124,#965,.T.);
#16808=EDGE_CURVE('',#13080,#13142,#966,.T.);
#16809=EDGE_CURVE('',#13140,#13100,#967,.T.);
#16810=EDGE_CURVE('',#13143,#13125,#968,.T.);
#16811=EDGE_CURVE('',#13142,#13143,#2546,.T.);
#16812=EDGE_CURVE('',#13101,#13139,#969,.T.);
#16813=EDGE_CURVE('',#13143,#13081,#970,.T.);
#16814=EDGE_CURVE('',#13081,#13144,#2547,.T.);
#16815=EDGE_CURVE('',#13144,#13080,#2548,.T.);
#16816=EDGE_CURVE('',#13145,#13145,#2549,.T.);
#16817=EDGE_CURVE('',#13144,#13145,#8267,.T.);
#23661=ORIENTED_EDGE('',*,*,#16714,.F.);
#23662=ORIENTED_EDGE('',*,*,#16715,.T.);
#23663=ORIENTED_EDGE('',*,*,#16716,.T.);
#23664=ORIENTED_EDGE('',*,*,#16717,.T.);
#23665=ORIENTED_EDGE('',*,*,#16718,.F.);
#23666=ORIENTED_EDGE('',*,*,#16719,.T.);
#23667=ORIENTED_EDGE('',*,*,#16714,.T.);
#23668=ORIENTED_EDGE('',*,*,#16720,.T.);
#23669=ORIENTED_EDGE('',*,*,#16721,.F.);
#23670=ORIENTED_EDGE('',*,*,#16722,.T.);
#23671=ORIENTED_EDGE('',*,*,#16718,.T.);
#23672=ORIENTED_EDGE('',*,*,#16723,.T.);
#23673=ORIENTED_EDGE('',*,*,#16724,.F.);
#23674=ORIENTED_EDGE('',*,*,#16725,.T.);
#23675=ORIENTED_EDGE('',*,*,#16721,.T.);
#23676=ORIENTED_EDGE('',*,*,#16726,.T.);
#23677=ORIENTED_EDGE('',*,*,#16727,.F.);
#23678=ORIENTED_EDGE('',*,*,#16728,.T.);
#23679=ORIENTED_EDGE('',*,*,#16724,.T.);
#23680=ORIENTED_EDGE('',*,*,#16729,.T.);
#23681=ORIENTED_EDGE('',*,*,#16730,.F.);
#23682=ORIENTED_EDGE('',*,*,#16731,.T.);
#23683=ORIENTED_EDGE('',*,*,#16727,.T.);
#23684=ORIENTED_EDGE('',*,*,#16732,.T.);
#23685=ORIENTED_EDGE('',*,*,#16733,.F.);
#23686=ORIENTED_EDGE('',*,*,#16734,.T.);
#23687=ORIENTED_EDGE('',*,*,#16730,.T.);
#23688=ORIENTED_EDGE('',*,*,#16735,.T.);
#23689=ORIENTED_EDGE('',*,*,#16736,.F.);
#23690=ORIENTED_EDGE('',*,*,#16737,.T.);
#23691=ORIENTED_EDGE('',*,*,#16733,.T.);
#23692=ORIENTED_EDGE('',*,*,#16738,.T.);
#23693=ORIENTED_EDGE('',*,*,#16739,.F.);
#23694=ORIENTED_EDGE('',*,*,#16740,.T.);
#23695=ORIENTED_EDGE('',*,*,#16736,.T.);
#23696=ORIENTED_EDGE('',*,*,#16741,.T.);
#23697=ORIENTED_EDGE('',*,*,#16742,.F.);
#23698=ORIENTED_EDGE('',*,*,#16743,.T.);
#23699=ORIENTED_EDGE('',*,*,#16739,.T.);
#23700=ORIENTED_EDGE('',*,*,#16744,.T.);
#23701=ORIENTED_EDGE('',*,*,#16745,.F.);
#23702=ORIENTED_EDGE('',*,*,#16746,.T.);
#23703=ORIENTED_EDGE('',*,*,#16742,.T.);
#23704=ORIENTED_EDGE('',*,*,#16747,.T.);
#23705=ORIENTED_EDGE('',*,*,#16748,.F.);
#23706=ORIENTED_EDGE('',*,*,#16749,.T.);
#23707=ORIENTED_EDGE('',*,*,#16750,.T.);
#23708=ORIENTED_EDGE('',*,*,#16751,.F.);
#23709=ORIENTED_EDGE('',*,*,#16752,.F.);
#23710=ORIENTED_EDGE('',*,*,#16753,.T.);
#23711=ORIENTED_EDGE('',*,*,#16748,.T.);
#23712=ORIENTED_EDGE('',*,*,#16754,.F.);
#23713=ORIENTED_EDGE('',*,*,#16755,.F.);
#23714=ORIENTED_EDGE('',*,*,#16756,.T.);
#23715=ORIENTED_EDGE('',*,*,#16752,.T.);
#23716=ORIENTED_EDGE('',*,*,#16757,.F.);
#23717=ORIENTED_EDGE('',*,*,#16758,.F.);
#23718=ORIENTED_EDGE('',*,*,#16759,.T.);
#23719=ORIENTED_EDGE('',*,*,#16755,.T.);
#23720=ORIENTED_EDGE('',*,*,#16760,.F.);
#23721=ORIENTED_EDGE('',*,*,#16761,.F.);
#23722=ORIENTED_EDGE('',*,*,#16762,.T.);
#23723=ORIENTED_EDGE('',*,*,#16758,.T.);
#23724=ORIENTED_EDGE('',*,*,#16763,.F.);
#23725=ORIENTED_EDGE('',*,*,#16764,.F.);
#23726=ORIENTED_EDGE('',*,*,#16765,.T.);
#23727=ORIENTED_EDGE('',*,*,#16761,.T.);
#23728=ORIENTED_EDGE('',*,*,#16766,.F.);
#23729=ORIENTED_EDGE('',*,*,#16767,.F.);
#23730=ORIENTED_EDGE('',*,*,#16768,.T.);
#23731=ORIENTED_EDGE('',*,*,#16764,.T.);
#23732=ORIENTED_EDGE('',*,*,#16769,.F.);
#23733=ORIENTED_EDGE('',*,*,#16770,.F.);
#23734=ORIENTED_EDGE('',*,*,#16771,.T.);
#23735=ORIENTED_EDGE('',*,*,#16767,.T.);
#23736=ORIENTED_EDGE('',*,*,#16772,.F.);
#23737=ORIENTED_EDGE('',*,*,#16773,.F.);
#23738=ORIENTED_EDGE('',*,*,#16774,.T.);
#23739=ORIENTED_EDGE('',*,*,#16770,.T.);
#23740=ORIENTED_EDGE('',*,*,#16775,.F.);
#23741=ORIENTED_EDGE('',*,*,#16776,.F.);
#23742=ORIENTED_EDGE('',*,*,#16777,.T.);
#23743=ORIENTED_EDGE('',*,*,#16773,.T.);
#23744=ORIENTED_EDGE('',*,*,#16778,.F.);
#23745=ORIENTED_EDGE('',*,*,#16779,.F.);
#23746=ORIENTED_EDGE('',*,*,#16780,.T.);
#23747=ORIENTED_EDGE('',*,*,#16776,.T.);
#23748=ORIENTED_EDGE('',*,*,#16781,.F.);
#23749=ORIENTED_EDGE('',*,*,#16782,.F.);
#23750=ORIENTED_EDGE('',*,*,#16783,.F.);
#23751=ORIENTED_EDGE('',*,*,#16784,.F.);
#23752=ORIENTED_EDGE('',*,*,#16785,.F.);
#23753=ORIENTED_EDGE('',*,*,#16786,.F.);
#23754=ORIENTED_EDGE('',*,*,#16787,.F.);
#23755=ORIENTED_EDGE('',*,*,#16788,.F.);
#23756=ORIENTED_EDGE('',*,*,#16789,.T.);
#23757=ORIENTED_EDGE('',*,*,#16788,.T.);
#23758=ORIENTED_EDGE('',*,*,#16790,.F.);
#23759=ORIENTED_EDGE('',*,*,#16791,.F.);
#23760=ORIENTED_EDGE('',*,*,#16792,.F.);
#23761=ORIENTED_EDGE('',*,*,#16793,.F.);
#23762=ORIENTED_EDGE('',*,*,#16794,.F.);
#23763=ORIENTED_EDGE('',*,*,#16782,.T.);
#23764=ORIENTED_EDGE('',*,*,#16789,.F.);
#23765=ORIENTED_EDGE('',*,*,#16795,.T.);
#23766=ORIENTED_EDGE('',*,*,#16785,.T.);
#23767=ORIENTED_EDGE('',*,*,#16796,.T.);
#23768=ORIENTED_EDGE('',*,*,#16792,.T.);
#23769=ORIENTED_EDGE('',*,*,#16797,.T.);
#23770=ORIENTED_EDGE('',*,*,#16783,.T.);
#23771=ORIENTED_EDGE('',*,*,#16794,.T.);
#23772=ORIENTED_EDGE('',*,*,#16798,.T.);
#23773=ORIENTED_EDGE('',*,*,#16784,.T.);
#23774=ORIENTED_EDGE('',*,*,#16798,.F.);
#23775=ORIENTED_EDGE('',*,*,#16793,.T.);
#23776=ORIENTED_EDGE('',*,*,#16796,.F.);
#23777=ORIENTED_EDGE('',*,*,#16786,.T.);
#23778=ORIENTED_EDGE('',*,*,#16797,.F.);
#23779=ORIENTED_EDGE('',*,*,#16791,.T.);
#23780=ORIENTED_EDGE('',*,*,#16799,.F.);
#23781=ORIENTED_EDGE('',*,*,#16790,.T.);
#23782=ORIENTED_EDGE('',*,*,#16787,.T.);
#23783=ORIENTED_EDGE('',*,*,#16799,.T.);
#23784=ORIENTED_EDGE('',*,*,#16800,.F.);
#23785=ORIENTED_EDGE('',*,*,#16801,.F.);
#23786=ORIENTED_EDGE('',*,*,#16750,.F.);
#23787=ORIENTED_EDGE('',*,*,#16802,.F.);
#23788=ORIENTED_EDGE('',*,*,#16803,.F.);
#23789=ORIENTED_EDGE('',*,*,#16804,.F.);
#23790=ORIENTED_EDGE('',*,*,#16805,.T.);
#23791=ORIENTED_EDGE('',*,*,#16800,.T.);
#23792=ORIENTED_EDGE('',*,*,#16805,.F.);
#23793=ORIENTED_EDGE('',*,*,#16795,.F.);
#23794=ORIENTED_EDGE('',*,*,#16806,.T.);
#23795=ORIENTED_EDGE('',*,*,#16804,.T.);
#23796=ORIENTED_EDGE('',*,*,#16806,.F.);
#23797=ORIENTED_EDGE('',*,*,#16802,.T.);
#23798=ORIENTED_EDGE('',*,*,#16749,.F.);
#23799=ORIENTED_EDGE('',*,*,#16753,.F.);
#23800=ORIENTED_EDGE('',*,*,#16756,.F.);
#23801=ORIENTED_EDGE('',*,*,#16759,.F.);
#23802=ORIENTED_EDGE('',*,*,#16762,.F.);
#23803=ORIENTED_EDGE('',*,*,#16765,.F.);
#23804=ORIENTED_EDGE('',*,*,#16768,.F.);
#23805=ORIENTED_EDGE('',*,*,#16771,.F.);
#23806=ORIENTED_EDGE('',*,*,#16774,.F.);
#23807=ORIENTED_EDGE('',*,*,#16777,.F.);
#23808=ORIENTED_EDGE('',*,*,#16780,.F.);
#23809=ORIENTED_EDGE('',*,*,#16807,.F.);
#23810=ORIENTED_EDGE('',*,*,#16808,.F.);
#23811=ORIENTED_EDGE('',*,*,#16715,.F.);
#23812=ORIENTED_EDGE('',*,*,#16719,.F.);
#23813=ORIENTED_EDGE('',*,*,#16722,.F.);
#23814=ORIENTED_EDGE('',*,*,#16725,.F.);
#23815=ORIENTED_EDGE('',*,*,#16728,.F.);
#23816=ORIENTED_EDGE('',*,*,#16731,.F.);
#23817=ORIENTED_EDGE('',*,*,#16734,.F.);
#23818=ORIENTED_EDGE('',*,*,#16737,.F.);
#23819=ORIENTED_EDGE('',*,*,#16740,.F.);
#23820=ORIENTED_EDGE('',*,*,#16743,.F.);
#23821=ORIENTED_EDGE('',*,*,#16746,.F.);
#23822=ORIENTED_EDGE('',*,*,#16809,.F.);
#23823=ORIENTED_EDGE('',*,*,#16779,.T.);
#23824=ORIENTED_EDGE('',*,*,#16810,.F.);
#23825=ORIENTED_EDGE('',*,*,#16811,.F.);
#23826=ORIENTED_EDGE('',*,*,#16807,.T.);
#23827=ORIENTED_EDGE('',*,*,#16801,.T.);
#23828=ORIENTED_EDGE('',*,*,#16812,.F.);
#23829=ORIENTED_EDGE('',*,*,#16747,.F.);
#23830=ORIENTED_EDGE('',*,*,#16744,.F.);
#23831=ORIENTED_EDGE('',*,*,#16741,.F.);
#23832=ORIENTED_EDGE('',*,*,#16738,.F.);
#23833=ORIENTED_EDGE('',*,*,#16735,.F.);
#23834=ORIENTED_EDGE('',*,*,#16732,.F.);
#23835=ORIENTED_EDGE('',*,*,#16729,.F.);
#23836=ORIENTED_EDGE('',*,*,#16726,.F.);
#23837=ORIENTED_EDGE('',*,*,#16723,.F.);
#23838=ORIENTED_EDGE('',*,*,#16720,.F.);
#23839=ORIENTED_EDGE('',*,*,#16717,.F.);
#23840=ORIENTED_EDGE('',*,*,#16813,.F.);
#23841=ORIENTED_EDGE('',*,*,#16810,.T.);
#23842=ORIENTED_EDGE('',*,*,#16781,.T.);
#23843=ORIENTED_EDGE('',*,*,#16778,.T.);
#23844=ORIENTED_EDGE('',*,*,#16775,.T.);
#23845=ORIENTED_EDGE('',*,*,#16772,.T.);
#23846=ORIENTED_EDGE('',*,*,#16769,.T.);
#23847=ORIENTED_EDGE('',*,*,#16766,.T.);
#23848=ORIENTED_EDGE('',*,*,#16763,.T.);
#23849=ORIENTED_EDGE('',*,*,#16760,.T.);
#23850=ORIENTED_EDGE('',*,*,#16757,.T.);
#23851=ORIENTED_EDGE('',*,*,#16754,.T.);
#23852=ORIENTED_EDGE('',*,*,#16751,.T.);
#23853=ORIENTED_EDGE('',*,*,#16814,.T.);
#23854=ORIENTED_EDGE('',*,*,#16815,.T.);
#23855=ORIENTED_EDGE('',*,*,#16808,.T.);
#23856=ORIENTED_EDGE('',*,*,#16811,.T.);
#23857=ORIENTED_EDGE('',*,*,#16813,.T.);
#23858=ORIENTED_EDGE('',*,*,#16816,.F.);
#23859=ORIENTED_EDGE('',*,*,#16814,.F.);
#23860=ORIENTED_EDGE('',*,*,#16716,.F.);
#23861=ORIENTED_EDGE('',*,*,#16815,.F.);
#23862=ORIENTED_EDGE('',*,*,#16817,.T.);
#23863=ORIENTED_EDGE('',*,*,#16816,.T.);
#23864=ORIENTED_EDGE('',*,*,#16817,.F.);
#23865=ORIENTED_EDGE('',*,*,#16745,.T.);
#23866=ORIENTED_EDGE('',*,*,#16812,.T.);
#23867=ORIENTED_EDGE('',*,*,#16803,.T.);
#23868=ORIENTED_EDGE('',*,*,#16809,.T.);
#26752=PLANE('',#30213);
#26753=PLANE('',#30217);
#26754=PLANE('',#30222);
#26755=PLANE('',#30223);
#26756=PLANE('',#30231);
#26757=PLANE('',#30234);
#27988=ADVANCED_FACE('',(#4080),#1684,.T.);
#27989=ADVANCED_FACE('',(#4081),#1685,.T.);
#27990=ADVANCED_FACE('',(#4082),#1686,.T.);
#27991=ADVANCED_FACE('',(#4083),#1687,.T.);
#27992=ADVANCED_FACE('',(#4084),#1688,.T.);
#27993=ADVANCED_FACE('',(#4085),#1689,.T.);
#27994=ADVANCED_FACE('',(#4086),#1690,.T.);
#27995=ADVANCED_FACE('',(#4087),#1691,.T.);
#27996=ADVANCED_FACE('',(#4088),#1692,.T.);
#27997=ADVANCED_FACE('',(#4089),#1693,.T.);
#27998=ADVANCED_FACE('',(#4090),#1694,.T.);
#27999=ADVANCED_FACE('',(#4091),#1695,.T.);
#28000=ADVANCED_FACE('',(#4092),#1696,.T.);
#28001=ADVANCED_FACE('',(#4093),#1697,.T.);
#28002=ADVANCED_FACE('',(#4094),#1698,.T.);
#28003=ADVANCED_FACE('',(#4095),#1699,.T.);
#28004=ADVANCED_FACE('',(#4096),#1700,.T.);
#28005=ADVANCED_FACE('',(#4097),#1701,.T.);
#28006=ADVANCED_FACE('',(#4098),#1702,.T.);
#28007=ADVANCED_FACE('',(#4099),#1703,.T.);
#28008=ADVANCED_FACE('',(#4100),#1704,.T.);
#28009=ADVANCED_FACE('',(#4101),#1705,.T.);
#28010=ADVANCED_FACE('',(#4102),#380,.T.);
#28011=ADVANCED_FACE('',(#4103,#1974),#26752,.T.);
#28012=ADVANCED_FACE('',(#4104),#26753,.T.);
#28013=ADVANCED_FACE('',(#4105),#2889,.T.);
#28014=ADVANCED_FACE('',(#4106),#2890,.T.);
#28015=ADVANCED_FACE('',(#4107),#26754,.T.);
#28016=ADVANCED_FACE('',(#4108,#1975),#26755,.T.);
#28017=ADVANCED_FACE('',(#4109),#1706,.T.);
#28018=ADVANCED_FACE('',(#4110),#2891,.T.);
#28019=ADVANCED_FACE('',(#4111),#1462,.F.);
#28020=ADVANCED_FACE('',(#4112),#1707,.T.);
#28021=ADVANCED_FACE('',(#4113),#1463,.F.);
#28022=ADVANCED_FACE('',(#4114),#26756,.T.);
#28023=ADVANCED_FACE('',(#4115),#26757,.T.);
#28024=ADVANCED_FACE('',(#4116),#2892,.T.);
#28025=ADVANCED_FACE('',(#4117),#1708,.T.);
#28471=CLOSED_SHELL('',(#27988,#27989,#27990,#27991,#27992,#27993,#27994,
#27995,#27996,#27997,#27998,#27999,#28000,#28001,#28002,#28003,#28004,#28005,
#28006,#28007,#28008,#28009,#28010,#28011,#28012,#28013,#28014,#28015,#28016,
#28017,#28018,#28019,#28020,#28021,#28022,#28023,#28024,#28025));
#30184=AXIS2_PLACEMENT_3D('',#56990,#35788,#35789);
#30185=AXIS2_PLACEMENT_3D('',#56991,#35790,#35791);
#30186=AXIS2_PLACEMENT_3D('',#57007,#35793,#35794);
#30187=AXIS2_PLACEMENT_3D('',#57018,#35795,#35796);
#30188=AXIS2_PLACEMENT_3D('',#57066,#35798,#35799);
#30189=AXIS2_PLACEMENT_3D('',#57114,#35801,#35802);
#30190=AXIS2_PLACEMENT_3D('',#57168,#35804,#35805);
#30191=AXIS2_PLACEMENT_3D('',#57216,#35807,#35808);
#30192=AXIS2_PLACEMENT_3D('',#57264,#35810,#35811);
#30193=AXIS2_PLACEMENT_3D('',#57318,#35813,#35814);
#30194=AXIS2_PLACEMENT_3D('',#57366,#35816,#35817);
#30195=AXIS2_PLACEMENT_3D('',#57414,#35819,#35820);
#30196=AXIS2_PLACEMENT_3D('',#57468,#35822,#35823);
#30197=AXIS2_PLACEMENT_3D('',#57516,#35825,#35826);
#30198=AXIS2_PLACEMENT_3D('',#57527,#35828,#35829);
#30199=AXIS2_PLACEMENT_3D('',#57532,#35830,#35831);
#30200=AXIS2_PLACEMENT_3D('',#57557,#35833,#35834);
#30201=AXIS2_PLACEMENT_3D('',#57582,#35836,#35837);
#30202=AXIS2_PLACEMENT_3D('',#57607,#35839,#35840);
#30203=AXIS2_PLACEMENT_3D('',#57631,#35842,#35843);
#30204=AXIS2_PLACEMENT_3D('',#57656,#35845,#35846);
#30205=AXIS2_PLACEMENT_3D('',#57681,#35848,#35849);
#30206=AXIS2_PLACEMENT_3D('',#57705,#35851,#35852);
#30207=AXIS2_PLACEMENT_3D('',#57730,#35854,#35855);
#30208=AXIS2_PLACEMENT_3D('',#57755,#35857,#35858);
#30209=AXIS2_PLACEMENT_3D('',#57779,#35860,#35861);
#30210=AXIS2_PLACEMENT_3D('',#57782,#35862,#35863);
#30211=AXIS2_PLACEMENT_3D('',#57838,#35864,#35865);
#30212=AXIS2_PLACEMENT_3D('',#57839,#35866,#35867);
#30213=AXIS2_PLACEMENT_3D('',#57894,#35868,#35869);
#30214=AXIS2_PLACEMENT_3D('',#57896,#35870,#35871);
#30215=AXIS2_PLACEMENT_3D('',#57897,#35872,#35873);
#30216=AXIS2_PLACEMENT_3D('',#57898,#35874,#35875);
#30217=AXIS2_PLACEMENT_3D('',#57899,#35876,#35877);
#30218=AXIS2_PLACEMENT_3D('',#57900,#35878,#35879);
#30219=AXIS2_PLACEMENT_3D('',#57901,#35880,#35881);
#30220=AXIS2_PLACEMENT_3D('',#57902,#35882,#35883);
#30221=AXIS2_PLACEMENT_3D('',#57903,#35884,#35885);
#30222=AXIS2_PLACEMENT_3D('',#57904,#35886,#35887);
#30223=AXIS2_PLACEMENT_3D('',#57905,#35888,#35889);
#30224=AXIS2_PLACEMENT_3D('',#57907,#35890,#35891);
#30225=AXIS2_PLACEMENT_3D('',#58044,#35892,#35893);
#30226=AXIS2_PLACEMENT_3D('',#58045,#35894,#35895);
#30227=AXIS2_PLACEMENT_3D('',#58047,#35896,#35897);
#30228=AXIS2_PLACEMENT_3D('',#58049,#35899,#35900);
#30229=AXIS2_PLACEMENT_3D('',#58448,#35902,#35903);
#30230=AXIS2_PLACEMENT_3D('',#58459,#35904,#35905);
#30231=AXIS2_PLACEMENT_3D('',#58844,#35906,#35907);
#30232=AXIS2_PLACEMENT_3D('',#58846,#35908,#35909);
#30233=AXIS2_PLACEMENT_3D('',#58847,#35910,#35911);
#30234=AXIS2_PLACEMENT_3D('',#58848,#35912,#35913);
#30235=AXIS2_PLACEMENT_3D('',#58850,#35914,#35915);
#30236=AXIS2_PLACEMENT_3D('',#58851,#35916,#35917);
#30237=AXIS2_PLACEMENT_3D('',#58853,#35919,#35920);
#35788=DIRECTION('axis',(0.,0.,1.));
#35789=DIRECTION('refdir',(1.,0.,0.));
#35790=DIRECTION('center_axis',(0.,0.,1.));
#35791=DIRECTION('ref_axis',(1.,0.,0.));
#35792=DIRECTION('',(0.,0.,-1.));
#35793=DIRECTION('center_axis',(0.,0.,1.));
#35794=DIRECTION('ref_axis',(1.,0.,0.));
#35795=DIRECTION('center_axis',(0.,0.,1.));
#35796=DIRECTION('ref_axis',(1.,0.,0.));
#35797=DIRECTION('',(0.,0.,-1.));
#35798=DIRECTION('center_axis',(0.,0.,1.));
#35799=DIRECTION('ref_axis',(1.,0.,0.));
#35800=DIRECTION('',(0.,0.,-1.));
#35801=DIRECTION('center_axis',(0.,0.,1.));
#35802=DIRECTION('ref_axis',(1.,0.,0.));
#35803=DIRECTION('',(0.,0.,-1.));
#35804=DIRECTION('center_axis',(0.,0.,1.));
#35805=DIRECTION('ref_axis',(1.,0.,0.));
#35806=DIRECTION('',(0.,0.,-1.));
#35807=DIRECTION('center_axis',(0.,0.,1.));
#35808=DIRECTION('ref_axis',(1.,0.,0.));
#35809=DIRECTION('',(0.,0.,-1.));
#35810=DIRECTION('center_axis',(0.,0.,1.));
#35811=DIRECTION('ref_axis',(1.,0.,0.));
#35812=DIRECTION('',(0.,0.,-1.));
#35813=DIRECTION('center_axis',(0.,0.,1.));
#35814=DIRECTION('ref_axis',(1.,0.,0.));
#35815=DIRECTION('',(0.,0.,-1.));
#35816=DIRECTION('center_axis',(0.,0.,1.));
#35817=DIRECTION('ref_axis',(1.,0.,0.));
#35818=DIRECTION('',(0.,0.,-1.));
#35819=DIRECTION('center_axis',(0.,0.,1.));
#35820=DIRECTION('ref_axis',(1.,0.,0.));
#35821=DIRECTION('',(0.,0.,-1.));
#35822=DIRECTION('center_axis',(0.,0.,1.));
#35823=DIRECTION('ref_axis',(1.,0.,0.));
#35824=DIRECTION('',(0.,0.,-1.));
#35825=DIRECTION('center_axis',(0.,0.,1.));
#35826=DIRECTION('ref_axis',(1.,5.61770717067589E-14,0.));
#35827=DIRECTION('',(0.,0.,1.));
#35828=DIRECTION('center_axis',(0.,0.,-1.));
#35829=DIRECTION('ref_axis',(1.,5.61770717067589E-14,0.));
#35830=DIRECTION('center_axis',(0.,0.,1.));
#35831=DIRECTION('ref_axis',(1.,5.61770717067589E-14,0.));
#35832=DIRECTION('',(0.,0.,1.));
#35833=DIRECTION('center_axis',(0.,0.,1.));
#35834=DIRECTION('ref_axis',(1.,5.61770717067589E-14,0.));
#35835=DIRECTION('',(0.,0.,1.));
#35836=DIRECTION('center_axis',(0.,0.,1.));
#35837=DIRECTION('ref_axis',(1.,5.61770717067589E-14,0.));
#35838=DIRECTION('',(0.,0.,1.));
#35839=DIRECTION('center_axis',(0.,0.,1.));
#35840=DIRECTION('ref_axis',(1.,5.61770717067589E-14,0.));
#35841=DIRECTION('',(0.,0.,1.));
#35842=DIRECTION('center_axis',(0.,0.,1.));
#35843=DIRECTION('ref_axis',(1.,5.61770717067589E-14,0.));
#35844=DIRECTION('',(0.,0.,1.));
#35845=DIRECTION('center_axis',(0.,0.,1.));
#35846=DIRECTION('ref_axis',(1.,5.61770717067589E-14,0.));
#35847=DIRECTION('',(0.,0.,1.));
#35848=DIRECTION('center_axis',(0.,0.,1.));
#35849=DIRECTION('ref_axis',(1.,5.61770717067589E-14,0.));
#35850=DIRECTION('',(0.,0.,1.));
#35851=DIRECTION('center_axis',(0.,0.,1.));
#35852=DIRECTION('ref_axis',(1.,5.61770717067589E-14,0.));
#35853=DIRECTION('',(0.,0.,1.));
#35854=DIRECTION('center_axis',(0.,0.,1.));
#35855=DIRECTION('ref_axis',(1.,5.61770717067589E-14,0.));
#35856=DIRECTION('',(0.,0.,1.));
#35857=DIRECTION('center_axis',(0.,0.,1.));
#35858=DIRECTION('ref_axis',(1.,5.61770717067589E-14,0.));
#35859=DIRECTION('',(0.,0.,1.));
#35860=DIRECTION('center_axis',(0.,1.,0.));
#35861=DIRECTION('ref_axis',(0.,0.,1.));
#35862=DIRECTION('center_axis',(-1.,0.,1.22464679914735E-16));
#35863=DIRECTION('ref_axis',(-1.22464679914735E-16,0.,-1.));
#35864=DIRECTION('center_axis',(-1.,0.,1.22464679914735E-16));
#35865=DIRECTION('ref_axis',(-1.22464679914735E-16,0.,-1.));
#35866=DIRECTION('center_axis',(0.,-1.,0.));
#35867=DIRECTION('ref_axis',(0.,0.,1.));
#35868=DIRECTION('center_axis',(0.,0.,1.));
#35869=DIRECTION('ref_axis',(1.,0.,0.));
#35870=DIRECTION('center_axis',(0.,0.,1.));
#35871=DIRECTION('ref_axis',(1.,0.,0.));
#35872=DIRECTION('center_axis',(0.,0.,-1.));
#35873=DIRECTION('ref_axis',(1.,0.,0.));
#35874=DIRECTION('center_axis',(0.,0.,-1.));
#35875=DIRECTION('ref_axis',(1.,0.,0.));
#35876=DIRECTION('center_axis',(0.,0.,1.));
#35877=DIRECTION('ref_axis',(1.,0.,0.));
#35878=DIRECTION('center_axis',(0.,0.,1.));
#35879=DIRECTION('ref_axis',(1.,0.,0.));
#35880=DIRECTION('center_axis',(0.,0.,-1.));
#35881=DIRECTION('ref_axis',(1.,0.,0.));
#35882=DIRECTION('center_axis',(0.,0.,-1.));
#35883=DIRECTION('ref_axis',(1.,0.,0.));
#35884=DIRECTION('center_axis',(0.,0.,1.));
#35885=DIRECTION('ref_axis',(1.,0.,0.));
#35886=DIRECTION('center_axis',(0.,0.,1.));
#35887=DIRECTION('ref_axis',(1.,0.,0.));
#35888=DIRECTION('center_axis',(0.,0.,-1.));
#35889=DIRECTION('ref_axis',(-1.,0.,0.));
#35890=DIRECTION('center_axis',(0.,0.,1.));
#35891=DIRECTION('ref_axis',(1.,0.,0.));
#35892=DIRECTION('center_axis',(0.,0.,-1.));
#35893=DIRECTION('ref_axis',(1.,0.,0.));
#35894=DIRECTION('center_axis',(0.,0.,1.));
#35895=DIRECTION('ref_axis',(1.,0.,0.));
#35896=DIRECTION('center_axis',(0.,0.,1.));
#35897=DIRECTION('ref_axis',(1.,0.,0.));
#35898=DIRECTION('',(0.,0.,-1.));
#35899=DIRECTION('center_axis',(0.,0.,-1.));
#35900=DIRECTION('ref_axis',(1.,0.,0.));
#35901=DIRECTION('',(-0.707106781186547,-8.65956056235493E-17,-0.707106781186548));
#35902=DIRECTION('center_axis',(0.,0.,1.));
#35903=DIRECTION('ref_axis',(1.,5.61770717067589E-14,0.));
#35904=DIRECTION('center_axis',(0.,0.,-1.));
#35905=DIRECTION('ref_axis',(1.,5.61770717067589E-14,0.));
#35906=DIRECTION('center_axis',(0.,0.,1.));
#35907=DIRECTION('ref_axis',(1.,0.,0.));
#35908=DIRECTION('center_axis',(0.,0.,1.));
#35909=DIRECTION('ref_axis',(1.,0.,0.));
#35910=DIRECTION('center_axis',(0.,0.,1.));
#35911=DIRECTION('ref_axis',(1.,0.,0.));
#35912=DIRECTION('center_axis',(0.,0.,-1.));
#35913=DIRECTION('ref_axis',(-1.,0.,0.));
#35914=DIRECTION('center_axis',(0.,0.,1.));
#35915=DIRECTION('ref_axis',(1.,0.,0.));
#35916=DIRECTION('center_axis',(0.,0.,1.));
#35917=DIRECTION('ref_axis',(1.,0.,0.));
#35918=DIRECTION('',(0.707106781186547,8.65956056235493E-17,-0.707106781186548));
#35919=DIRECTION('center_axis',(0.,0.,1.));
#35920=DIRECTION('ref_axis',(1.,0.,0.));
#56990=CARTESIAN_POINT('',(0.,0.,0.));
#56991=CARTESIAN_POINT('Origin',(0.,0.,-0.785));
#56992=CARTESIAN_POINT('',(-0.492894796571446,0.000311056548144339,-1.57911584740964));
#56993=CARTESIAN_POINT('',(-0.492681024549354,0.000145720506528142,-1.60088415259036));
#56994=CARTESIAN_POINT('',(-0.4925,-6.03138548580071E-17,-0.785));
#56995=CARTESIAN_POINT('',(0.217165055346613,0.442373225884384,-1.6275));
#56996=CARTESIAN_POINT('Ctrl Pts',(-0.492894796571446,0.000311056548144339,
-1.57911584740964));
#56997=CARTESIAN_POINT('Ctrl Pts',(-0.493072781975635,0.0225970133474953,
-1.58019890716347));
#56998=CARTESIAN_POINT('Ctrl Pts',(-0.49169270506612,0.0448619688323287,
-1.58128196691731));
#56999=CARTESIAN_POINT('Ctrl Pts',(-0.48867934824822,0.0669043084087307,
-1.58236502667114));
#57000=CARTESIAN_POINT('Ctrl Pts',(-0.46677608813157,0.227123999105002,
-1.5902374894904));
#57001=CARTESIAN_POINT('Ctrl Pts',(-0.358579539374524,0.375581922119211,
-1.59810995230966));
#57002=CARTESIAN_POINT('Ctrl Pts',(-0.212592472031373,0.445197883180087,
-1.60598241512892));
#57003=CARTESIAN_POINT('Ctrl Pts',(-0.0795850009787494,0.508624343442078,
-1.61315494341928));
#57004=CARTESIAN_POINT('Ctrl Pts',(0.0847918659550201,0.50660516259901,
-1.62032747170964));
#57005=CARTESIAN_POINT('Ctrl Pts',(0.217490523462166,0.442550970777087,
-1.6275));
#57006=CARTESIAN_POINT('',(-0.21683958723106,0.44219548099168,-1.6275));
#57007=CARTESIAN_POINT('Origin',(0.,0.,-1.6275));
#57008=CARTESIAN_POINT('Ctrl Pts',(-0.216839587231058,0.442195480991681,
-1.6275));
#57009=CARTESIAN_POINT('Ctrl Pts',(-0.289748988500098,0.406442866693165,
-1.62356376859037));
#57010=CARTESIAN_POINT('Ctrl Pts',(-0.353117841415619,0.352318189275016,
-1.61962753718074));
#57011=CARTESIAN_POINT('Ctrl Pts',(-0.400486606282593,0.286264167711519,
-1.61569130577111));
#57012=CARTESIAN_POINT('Ctrl Pts',(-0.447855371149569,0.220210146148021,
-1.61175507436148));
#57013=CARTESIAN_POINT('Ctrl Pts',(-0.479224047967998,0.142226780439174,
-1.60781884295185));
#57014=CARTESIAN_POINT('Ctrl Pts',(-0.489180114775594,0.0617636412371016,
-1.60388261154222));
#57015=CARTESIAN_POINT('Ctrl Pts',(-0.491708155307928,0.0413324728658215,
-1.60288312522493));
#57016=CARTESIAN_POINT('Ctrl Pts',(-0.49285561428007,0.0207414206897894,
-1.60188363890765));
#57017=CARTESIAN_POINT('Ctrl Pts',(-0.492681024549354,0.000145720506528142,
-1.60088415259036));
#57018=CARTESIAN_POINT('Origin',(0.,0.,-0.785));
#57019=CARTESIAN_POINT('',(-0.491724062797573,2.84481552980109E-5,-1.42911584740964));
#57020=CARTESIAN_POINT('',(-0.491725215890323,5.26094410910955E-5,-1.45088415259036));
#57021=CARTESIAN_POINT('',(-0.4925,-6.03138548580071E-17,-0.785));
#57022=CARTESIAN_POINT('Ctrl Pts',(-0.491724062797573,2.84481552980109E-5,
-1.42911584740964));
#57023=CARTESIAN_POINT('Ctrl Pts',(-0.491766038698159,0.0797124417823624,
-1.43296413024792));
#57024=CARTESIAN_POINT('Ctrl Pts',(-0.473465280791214,0.159378202380034,
-1.43681241308619));
#57025=CARTESIAN_POINT('Ctrl Pts',(-0.43671528821848,0.229354820363482,
-1.44066069592447));
#57026=CARTESIAN_POINT('Ctrl Pts',(-0.361535536028939,0.372506544507255,
-1.44853315874373));
#57027=CARTESIAN_POINT('Ctrl Pts',(-0.209147193490587,0.475109971852566,
-1.45640562156299));
#57028=CARTESIAN_POINT('Ctrl Pts',(-0.048228220013445,0.490917381779544,
-1.46427808438225));
#57029=CARTESIAN_POINT('Ctrl Pts',(0.112690753463697,0.506724791706522,
-1.47215054720151));
#57030=CARTESIAN_POINT('Ctrl Pts',(0.282140357879629,0.435736184215168,
-1.48002301002077));
#57031=CARTESIAN_POINT('Ctrl Pts',(0.383738024817693,0.309953148400658,
-1.48789547284003));
#57032=CARTESIAN_POINT('Ctrl Pts',(0.485335691755757,0.184170112586147,
-1.49576793565929));
#57033=CARTESIAN_POINT('Ctrl Pts',(0.519081421215954,0.00359264844848062,
-1.50364039847855));
#57034=CARTESIAN_POINT('Ctrl Pts',(0.469784530510368,-0.150403090698195,
-1.51151286129781));
#57035=CARTESIAN_POINT('Ctrl Pts',(0.420487639804781,-0.304398829844871,
-1.51938532411706));
#57036=CARTESIAN_POINT('Ctrl Pts',(0.288148128933412,-0.431812844000556,
-1.52725778693632));
#57037=CARTESIAN_POINT('Ctrl Pts',(0.132376511934491,-0.475195091226392,
-1.53513024975558));
#57038=CARTESIAN_POINT('Ctrl Pts',(-0.0233951050644308,-0.518577338452229,
-1.54300271257484));
#57039=CARTESIAN_POINT('Ctrl Pts',(-0.202598828190905,-0.477927818748217,
-1.5508751753941));
#57040=CARTESIAN_POINT('Ctrl Pts',(-0.324395704016015,-0.371612329707044,
-1.55874763821336));
#57041=CARTESIAN_POINT('Ctrl Pts',(-0.429436286749963,-0.27992327079748,
-1.56553704127879));
#57042=CARTESIAN_POINT('Ctrl Pts',(-0.491779055131949,-0.139393463792468,
-1.57232644434422));
#57043=CARTESIAN_POINT('Ctrl Pts',(-0.492894796571446,0.000311056548144339,
-1.57911584740964));
#57044=CARTESIAN_POINT('Ctrl Pts',(-0.492681024549354,0.000145720506528142,
-1.60088415259036));
#57045=CARTESIAN_POINT('Ctrl Pts',(-0.491480456721719,-0.141480793986821,
-1.59401117608839));
#57046=CARTESIAN_POINT('Ctrl Pts',(-0.427764999610373,-0.283327095887921,
-1.58713819958642));
#57047=CARTESIAN_POINT('Ctrl Pts',(-0.320567499630029,-0.374915910947789,
-1.58026522308444));
#57048=CARTESIAN_POINT('Ctrl Pts',(-0.197781057297411,-0.479823812351491,
-1.57239276026518));
#57049=CARTESIAN_POINT('Ctrl Pts',(-0.0179464790603139,-0.51879424278185,
-1.56452029744593));
#57050=CARTESIAN_POINT('Ctrl Pts',(0.137413483204638,-0.473829273326357,
-1.55664783462667));
#57051=CARTESIAN_POINT('Ctrl Pts',(0.29277344546959,-0.428864303870864,
-1.54877537180741));
#57052=CARTESIAN_POINT('Ctrl Pts',(0.423658791762397,-0.299963934529519,
-1.54090290898815));
#57053=CARTESIAN_POINT('Ctrl Pts',(0.471309471097307,-0.145433967873361,
-1.53303044616889));
#57054=CARTESIAN_POINT('Ctrl Pts',(0.518960150432216,0.00909599878279682,
-1.52515798334963));
#57055=CARTESIAN_POINT('Ctrl Pts',(0.483376162809228,0.189255562753767,
-1.51728552053037));
#57056=CARTESIAN_POINT('Ctrl Pts',(0.380476665429358,0.313951811038567,
-1.50941305771111));
#57057=CARTESIAN_POINT('Ctrl Pts',(0.277577168049488,0.438648059323367,
-1.50154059489185));
#57058=CARTESIAN_POINT('Ctrl Pts',(0.107362160912737,0.507880991921996,
-1.49366813207259));
#57059=CARTESIAN_POINT('Ctrl Pts',(-0.0533889325663778,0.490391165225274,
-1.48579566925333));
#57060=CARTESIAN_POINT('Ctrl Pts',(-0.214140026045492,0.472901338528552,
-1.47792320643407));
#57061=CARTESIAN_POINT('Ctrl Pts',(-0.365427205866971,0.368688752536479,
-1.47005074361481));
#57062=CARTESIAN_POINT('Ctrl Pts',(-0.439095781953566,0.224751935185655,
-1.46217828079555));
#57063=CARTESIAN_POINT('Ctrl Pts',(-0.474325009118265,0.155919563159685,
-1.45841357139382));
#57064=CARTESIAN_POINT('Ctrl Pts',(-0.491803862332235,0.0780027715797182,
-1.45464886199209));
#57065=CARTESIAN_POINT('Ctrl Pts',(-0.491725215890323,5.26094410910955E-5,
-1.45088415259036));
#57066=CARTESIAN_POINT('Origin',(0.,0.,-0.785));
#57067=CARTESIAN_POINT('',(-0.492844994071537,-0.000375497391989388,-1.27911584740964));
#57068=CARTESIAN_POINT('',(-0.492796742099722,-0.000388985907888563,-1.30088415259036));
#57069=CARTESIAN_POINT('',(-0.4925,-6.03138548580071E-17,-0.785));
#57070=CARTESIAN_POINT('Ctrl Pts',(-0.492844994071537,-0.000375497391989388,
-1.27911584740964));
#57071=CARTESIAN_POINT('Ctrl Pts',(-0.49169234062138,0.135775279584172,
-1.28572935333236));
#57072=CARTESIAN_POINT('Ctrl Pts',(-0.432845290990704,0.272801628077903,
-1.29234285925508));
#57073=CARTESIAN_POINT('Ctrl Pts',(-0.33250996431107,0.364365032885267,
-1.2989563651778));
#57074=CARTESIAN_POINT('Ctrl Pts',(-0.213074654511156,0.473358584622236,
-1.30682882799706));
#57075=CARTESIAN_POINT('Ctrl Pts',(-0.0348520950583099,0.517932941093665,
-1.31470129081632));
#57076=CARTESIAN_POINT('Ctrl Pts',(0.121830995151941,0.477997897412073,
-1.32257375363558));
#57077=CARTESIAN_POINT('Ctrl Pts',(0.278514085362191,0.438062853730481,
-1.33044621645484));
#57078=CARTESIAN_POINT('Ctrl Pts',(0.413657706329846,0.313618409895869,
-1.3383186792741));
#57079=CARTESIAN_POINT('Ctrl Pts',(0.466350984614939,0.160753135356507,
-1.34619114209336));
#57080=CARTESIAN_POINT('Ctrl Pts',(0.519044262900032,0.00788786081714538,
-1.35406360491262));
#57081=CARTESIAN_POINT('Ctrl Pts',(0.489287198502561,-0.173398244426965,
-1.36193606773188));
#57082=CARTESIAN_POINT('Ctrl Pts',(0.390491992071155,-0.301397825554306,
-1.36980853055114));
#57083=CARTESIAN_POINT('Ctrl Pts',(0.291696785639748,-0.429397406681647,
-1.3776809933704));
#57084=CARTESIAN_POINT('Ctrl Pts',(0.123863437174404,-0.504110463692217,
-1.38555345618966));
#57085=CARTESIAN_POINT('Ctrl Pts',(-0.0373644791913577,-0.491862563024499,
-1.39342591900891));
#57086=CARTESIAN_POINT('Ctrl Pts',(-0.198592395557119,-0.479614662356781,
-1.40129838182817));
#57087=CARTESIAN_POINT('Ctrl Pts',(-0.353214879823299,-0.380405804010775,
-1.40917084464743));
#57088=CARTESIAN_POINT('Ctrl Pts',(-0.431540541036024,-0.238951364366653,
-1.41704330746669));
#57089=CARTESIAN_POINT('Ctrl Pts',(-0.471578400227735,-0.166643861961637,
-1.42106748744768));
#57090=CARTESIAN_POINT('Ctrl Pts',(-0.49168016826437,-0.0832977379475879,
-1.42509166742866));
#57091=CARTESIAN_POINT('Ctrl Pts',(-0.491724062797573,2.84481552980109E-5,
-1.42911584740964));
#57092=CARTESIAN_POINT('Ctrl Pts',(-0.491725215890323,5.26094410910955E-5,
-1.45088415259036));
#57093=CARTESIAN_POINT('Ctrl Pts',(-0.491639403107431,-0.0850004479807165,
-1.44677639917283));
#57094=CARTESIAN_POINT('Ctrl Pts',(-0.470650596961721,-0.170093234554161,
-1.4426686457553));
#57095=CARTESIAN_POINT('Ctrl Pts',(-0.429009346683205,-0.24346817854896,
-1.43856089233777));
#57096=CARTESIAN_POINT('Ctrl Pts',(-0.349204362974535,-0.384090426223178,
-1.43068842951851));
#57097=CARTESIAN_POINT('Ctrl Pts',(-0.19354442320548,-0.481673872862038,
-1.42281596669926));
#57098=CARTESIAN_POINT('Ctrl Pts',(-0.0321958015858799,-0.492228826589368,
-1.41494350388));
#57099=CARTESIAN_POINT('Ctrl Pts',(0.12915282003372,-0.502783780316697,
-1.40707104106074));
#57100=CARTESIAN_POINT('Ctrl Pts',(0.296190123503867,-0.426310241132496,
-1.39919857824148));
#57101=CARTESIAN_POINT('Ctrl Pts',(0.393635112256126,-0.297279702079536,
-1.39132611542222));
#57102=CARTESIAN_POINT('Ctrl Pts',(0.491080101008387,-0.168249163026577,
-1.38345365260296));
#57103=CARTESIAN_POINT('Ctrl Pts',(0.51893277504276,0.0133383758951397,
-1.3755811897837));
#57104=CARTESIAN_POINT('Ctrl Pts',(0.464637291129985,0.165641568032344,
-1.36770872696444));
#57105=CARTESIAN_POINT('Ctrl Pts',(0.41034180721721,0.317944760169548,-1.35983626414518));
#57106=CARTESIAN_POINT('Ctrl Pts',(0.273898165357287,0.440963605522239,
-1.35196380132592));
#57107=CARTESIAN_POINT('Ctrl Pts',(0.116804197737899,0.479251095989714,
-1.34409133850666));
#57108=CARTESIAN_POINT('Ctrl Pts',(-0.0402897698814872,0.517538586457189,
-1.3362188756874));
#57109=CARTESIAN_POINT('Ctrl Pts',(-0.218034063260338,0.47109472203945,
-1.32834641286814));
#57110=CARTESIAN_POINT('Ctrl Pts',(-0.336318056393163,0.360852819953089,
-1.32047395004888));
#57111=CARTESIAN_POINT('Ctrl Pts',(-0.434430490466894,0.269411019045462,
-1.31394401756271));
#57112=CARTESIAN_POINT('Ctrl Pts',(-0.4916335119489,0.134075389234701,-1.30741408507653));
#57113=CARTESIAN_POINT('Ctrl Pts',(-0.492796742099722,-0.000388985907888563,
-1.30088415259036));
#57114=CARTESIAN_POINT('Origin',(0.,0.,-0.785));
#57115=CARTESIAN_POINT('',(-0.492699669112094,0.000410100521544665,-1.12911584740964));
#57116=CARTESIAN_POINT('',(-0.492749550373132,0.00040022685197263,-1.15088415259036));
#57117=CARTESIAN_POINT('',(-0.4925,-6.03138548580071E-17,-0.785));
#57118=CARTESIAN_POINT('Ctrl Pts',(-0.492699669112094,0.000410100521544665,
-1.12911584740964));
#57119=CARTESIAN_POINT('Ctrl Pts',(-0.49297563193663,0.0314429855949232,
-1.13062211359755));
#57120=CARTESIAN_POINT('Ctrl Pts',(-0.490290307645473,0.062428299335654,
-1.13212837978545));
#57121=CARTESIAN_POINT('Ctrl Pts',(-0.484469335446466,0.0928128968948493,
-1.13363464597335));
#57122=CARTESIAN_POINT('Ctrl Pts',(-0.454046168826502,0.25161724136183,
-1.14150710879261));
#57123=CARTESIAN_POINT('Ctrl Pts',(-0.337969510299702,0.39401239700866,
-1.14937957161187));
#57124=CARTESIAN_POINT('Ctrl Pts',(-0.188556356186219,0.455819340204937,
-1.15725203443113));
#57125=CARTESIAN_POINT('Ctrl Pts',(-0.039143202072734,0.517626283401215,
-1.16512449725039));
#57126=CARTESIAN_POINT('Ctrl Pts',(0.143606447627436,0.498845014146939,
-1.17299696006965));
#57127=CARTESIAN_POINT('Ctrl Pts',(0.277325367211442,0.407940450716456,
-1.18086942288891));
#57128=CARTESIAN_POINT('Ctrl Pts',(0.411044286795446,0.317035887285973,
-1.18874188570817));
#57129=CARTESIAN_POINT('Ctrl Pts',(0.495732476263288,0.154008029679284,
-1.19661434852743));
#57130=CARTESIAN_POINT('Ctrl Pts',(0.493220056252468,-0.00766471525244823,
-1.20448681134669));
#57131=CARTESIAN_POINT('Ctrl Pts',(0.490707636241647,-0.169337460184181,
-1.21235927416595));
#57132=CARTESIAN_POINT('Ctrl Pts',(0.400994606752165,-0.329655092440956,
-1.22023173698521));
#57133=CARTESIAN_POINT('Ctrl Pts',(0.26451559998051,-0.416360739939686,
-1.22810419980447));
#57134=CARTESIAN_POINT('Ctrl Pts',(0.128036593208856,-0.503066387438416,
-1.23597666262373));
#57135=CARTESIAN_POINT('Ctrl Pts',(-0.0552083908449711,-0.516160050179099,
-1.24384912544299));
#57136=CARTESIAN_POINT('Ctrl Pts',(-0.20262888612291,-0.449740264872263,
-1.25172158826224));
#57137=CARTESIAN_POINT('Ctrl Pts',(-0.350049381400848,-0.383320479565428,
-1.2595940510815));
#57138=CARTESIAN_POINT('Ctrl Pts',(-0.461645387902899,-0.237387246211074,
-1.26746651390076));
#57139=CARTESIAN_POINT('Ctrl Pts',(-0.487119361080433,-0.0777142560326435,
-1.27533897672002));
#57140=CARTESIAN_POINT('Ctrl Pts',(-0.49119313506329,-0.0521795006719227,
-1.27659793361656));
#57141=CARTESIAN_POINT('Ctrl Pts',(-0.493064414909343,-0.0262933632934072,
-1.2778568905131));
#57142=CARTESIAN_POINT('Ctrl Pts',(-0.492844994071537,-0.000375497391989388,
-1.27911584740964));
#57143=CARTESIAN_POINT('Ctrl Pts',(-0.492796742099722,-0.000388985907888563,
-1.30088415259036));
#57144=CARTESIAN_POINT('Ctrl Pts',(-0.493035897981524,-0.0280343716343784,
-1.29954162225727));
#57145=CARTESIAN_POINT('Ctrl Pts',(-0.490906259607873,-0.0556429295461318,
-1.29819909192419));
#57146=CARTESIAN_POINT('Ctrl Pts',(-0.486276335973135,-0.0828256273553652,
-1.2968565615911));
#57147=CARTESIAN_POINT('Ctrl Pts',(-0.45912692953348,-0.242222232822471,
-1.28898409877185));
#57148=CARTESIAN_POINT('Ctrl Pts',(-0.346004423767372,-0.386975504001697,
-1.28111163595259));
#57149=CARTESIAN_POINT('Ctrl Pts',(-0.197894517027637,-0.45184343470324,
-1.27323917313333));
#57150=CARTESIAN_POINT('Ctrl Pts',(-0.0497846102879024,-0.516711365404783,
-1.26536671031407));
#57151=CARTESIAN_POINT('Ctrl Pts',(0.13331269742546,-0.501693955628644,
-1.25749424749481));
#57152=CARTESIAN_POINT('Ctrl Pts',(0.268873574359746,-0.413559793115497,
-1.24962178467555));
#57153=CARTESIAN_POINT('Ctrl Pts',(0.404434451294034,-0.32542563060235,
-1.24174932185629));
#57154=CARTESIAN_POINT('Ctrl Pts',(0.492458897449246,-0.164174715352196,
-1.23387685903703));
#57155=CARTESIAN_POINT('Ctrl Pts',(0.493273304253071,-0.00248452317121441,
-1.22600439621777));
#57156=CARTESIAN_POINT('Ctrl Pts',(0.494087711056895,0.159205669009766,
-1.21813193339851));
#57157=CARTESIAN_POINT('Ctrl Pts',(0.407692078509334,0.321335138121573,
-1.21025947057925));
#57158=CARTESIAN_POINT('Ctrl Pts',(0.273025869168142,0.410830371438833,
-1.20238700775999));
#57159=CARTESIAN_POINT('Ctrl Pts',(0.138359659826949,0.500325604756093,
-1.19451454494073));
#57160=CARTESIAN_POINT('Ctrl Pts',(-0.0445771263078751,0.517186602278804,
-1.18664208212147));
#57161=CARTESIAN_POINT('Ctrl Pts',(-0.193332929681909,0.453813942791155,
-1.17876961930221));
#57162=CARTESIAN_POINT('Ctrl Pts',(-0.342088733055942,0.390441283303506,
-1.17089715648295));
#57163=CARTESIAN_POINT('Ctrl Pts',(-0.456663553669186,0.246834966805496,
-1.1630246936637));
#57164=CARTESIAN_POINT('Ctrl Pts',(-0.485417284176169,0.0877198949225954,
-1.15515223084444));
#57165=CARTESIAN_POINT('Ctrl Pts',(-0.490613589945532,0.0589649976818075,
-1.15372953809308));
#57166=CARTESIAN_POINT('Ctrl Pts',(-0.493007076876324,0.0297036021933078,
-1.15230684534172));
#57167=CARTESIAN_POINT('Ctrl Pts',(-0.492749550373132,0.00040022685197263,
-1.15088415259036));
#57168=CARTESIAN_POINT('Origin',(0.,0.,-0.785));
#57169=CARTESIAN_POINT('',(-0.491746356789813,-0.00010883115493171,-0.979115847409641));
#57170=CARTESIAN_POINT('',(-0.491736157223136,-8.20785977434006E-5,-1.00088415259036));
#57171=CARTESIAN_POINT('',(-0.4925,-6.03138548580071E-17,-0.785));
#57172=CARTESIAN_POINT('Ctrl Pts',(-0.491746356789813,-0.00010883115493171,
-0.979115847409641));
#57173=CARTESIAN_POINT('Ctrl Pts',(-0.491568688029523,0.0883286966854865,
-0.983387336681989));
#57174=CARTESIAN_POINT('Ctrl Pts',(-0.468769837714688,0.176851663470972,
-0.987658825954337));
#57175=CARTESIAN_POINT('Ctrl Pts',(-0.42390686631858,0.252245395083429,
-0.991930315226685));
#57176=CARTESIAN_POINT('Ctrl Pts',(-0.341223274775056,0.391197950288614,
-0.999802778045945));
#57177=CARTESIAN_POINT('Ctrl Pts',(-0.183593550391466,0.485553877341615,
-1.0076752408652));
#57178=CARTESIAN_POINT('Ctrl Pts',(-0.0220631010459361,0.492785947666456,
-1.01554770368446));
#57179=CARTESIAN_POINT('Ctrl Pts',(0.139467348299593,0.500018017991297,
-1.02342016650372));
#57180=CARTESIAN_POINT('Ctrl Pts',(0.304898522607063,0.420126231587979,
-1.03129262932298));
#57181=CARTESIAN_POINT('Ctrl Pts',(0.39966881688194,0.289118673655937,-1.03916509214224));
#57182=CARTESIAN_POINT('Ctrl Pts',(0.494439111156818,0.158111115723894,
-1.0470375549615));
#57183=CARTESIAN_POINT('Ctrl Pts',(0.518548525399102,-0.0240122137368738,
-1.05491001778076));
#57184=CARTESIAN_POINT('Ctrl Pts',(0.461130687884588,-0.17516637624073,
-1.06278248060002));
#57185=CARTESIAN_POINT('Ctrl Pts',(0.403712850370075,-0.326320538744583,
-1.07065494341928));
#57186=CARTESIAN_POINT('Ctrl Pts',(0.264767761098766,-0.446505534291526,
-1.07852740623854));
#57187=CARTESIAN_POINT('Ctrl Pts',(0.10691946257642,-0.481552696116318,
-1.0863998690578));
#57188=CARTESIAN_POINT('Ctrl Pts',(-0.0509288359459257,-0.51659985794111,
-1.09427233187706));
#57189=CARTESIAN_POINT('Ctrl Pts',(-0.227680343719308,-0.466509186043751,
-1.10214479469632));
#57190=CARTESIAN_POINT('Ctrl Pts',(-0.343671260249434,-0.353857083451506,
-1.11001725751558));
#57191=CARTESIAN_POINT('Ctrl Pts',(-0.437469223991527,-0.262759106553689,
-1.11638345414693));
#57192=CARTESIAN_POINT('Ctrl Pts',(-0.491533319088407,-0.130749617463121,
-1.12274965077829));
#57193=CARTESIAN_POINT('Ctrl Pts',(-0.492699669112094,0.000410100521544665,
-1.12911584740964));
#57194=CARTESIAN_POINT('Ctrl Pts',(-0.492749550373132,0.00040022685197263,
-1.15088415259036));
#57195=CARTESIAN_POINT('Ctrl Pts',(-0.4915820553322,-0.132446470359704,
-1.14443438252246));
#57196=CARTESIAN_POINT('Ctrl Pts',(-0.435929409661543,-0.266155961616792,
-1.13798461245456));
#57197=CARTESIAN_POINT('Ctrl Pts',(-0.339936079966906,-0.357446751494053,
-1.13153484238666));
#57198=CARTESIAN_POINT('Ctrl Pts',(-0.222768504849936,-0.468874498760009,
-1.1236623795674));
#57199=CARTESIAN_POINT('Ctrl Pts',(-0.0455007142152706,-0.517106166024128,
-1.11578991674814));
#57200=CARTESIAN_POINT('Ctrl Pts',(0.111970798701792,-0.480403224995691,
-1.10791745392888));
#57201=CARTESIAN_POINT('Ctrl Pts',(0.269442311618853,-0.443700283967254,
-1.10004499110962));
#57202=CARTESIAN_POINT('Ctrl Pts',(0.407117546818311,-0.322062734646261,
-1.09217252829036));
#57203=CARTESIAN_POINT('Ctrl Pts',(0.462944797876401,-0.17031392463671,
-1.0843000654711));
#57204=CARTESIAN_POINT('Ctrl Pts',(0.518772048934492,-0.0185651146271575,
-1.07642760265184));
#57205=CARTESIAN_POINT('Ctrl Pts',(0.492751315851212,0.163294956070952,
-1.06855513983258));
#57206=CARTESIAN_POINT('Ctrl Pts',(0.396610422658507,0.293300002140747,
-1.06068267701332));
#57207=CARTESIAN_POINT('Ctrl Pts',(0.300469529465803,0.423305048210542,
-1.05281021419406));
#57208=CARTESIAN_POINT('Ctrl Pts',(0.134208476163673,0.501455069652022,
-1.0449377513748));
#57209=CARTESIAN_POINT('Ctrl Pts',(-0.0272370970959901,0.49252701361753,
-1.03706528855555));
#57210=CARTESIAN_POINT('Ctrl Pts',(-0.188682670355654,0.483598957583038,
-1.02919282573629));
#57211=CARTESIAN_POINT('Ctrl Pts',(-0.345312763572852,0.387592824072574,
-1.02132036291703));
#57212=CARTESIAN_POINT('Ctrl Pts',(-0.426532513251872,0.247779607313462,
-1.01344790009777));
#57213=CARTESIAN_POINT('Ctrl Pts',(-0.469739001954307,0.173403138606935,
-1.00925998426196));
#57214=CARTESIAN_POINT('Ctrl Pts',(-0.491604942376349,0.0866296016571418,
-1.00507206842616));
#57215=CARTESIAN_POINT('Ctrl Pts',(-0.491736157223136,-8.20785977434006E-5,
-1.00088415259036));
#57216=CARTESIAN_POINT('Origin',(0.,0.,-0.785));
#57217=CARTESIAN_POINT('',(-0.493065289251647,-0.000280683390702752,-0.829115847409641));
#57218=CARTESIAN_POINT('',(-0.493025735351581,-0.000302692969106977,-0.850884152590359));
#57219=CARTESIAN_POINT('',(-0.4925,-6.03138548580071E-17,-0.785));
#57220=CARTESIAN_POINT('Ctrl Pts',(-0.493065289251647,-0.000280683390702752,
-0.829115847409641));
#57221=CARTESIAN_POINT('Ctrl Pts',(-0.492073025151649,0.144413259987423,
-0.836152559766433));
#57222=CARTESIAN_POINT('Ctrl Pts',(-0.424455104245118,0.289914875416531,
-0.843189272123224));
#57223=CARTESIAN_POINT('Ctrl Pts',(-0.31267145716183,0.38152500642237,-0.850225984480016));
#57224=CARTESIAN_POINT('Ctrl Pts',(-0.187611264156348,0.484015674456412,
-0.858098447299275));
#57225=CARTESIAN_POINT('Ctrl Pts',(-0.00727120091729211,0.519053262387343,
-0.865970910118535));
#57226=CARTESIAN_POINT('Ctrl Pts',(0.147067531334825,0.470845953445812,
-0.873843372937794));
#57227=CARTESIAN_POINT('Ctrl Pts',(0.301406263586942,0.422638644504282,
-0.881715835757054));
#57228=CARTESIAN_POINT('Ctrl Pts',(0.429743664852121,0.29118643869029,-0.889588298576313));
#57229=CARTESIAN_POINT('Ctrl Pts',(0.474236691555723,0.135736255404997,
-0.897460761395573));
#57230=CARTESIAN_POINT('Ctrl Pts',(0.518729718259325,-0.0197139278802952,
-0.905333224214832));
#57231=CARTESIAN_POINT('Ctrl Pts',(0.479378370401352,-0.199162088636888,
-0.913205687034091));
#57232=CARTESIAN_POINT('Ctrl Pts',(0.373918722627788,-0.321729015660929,
-0.921078149853351));
#57233=CARTESIAN_POINT('Ctrl Pts',(0.268459074854222,-0.444295942684971,
-0.92895061267261));
#57234=CARTESIAN_POINT('Ctrl Pts',(0.0968911271650634,-0.509981635976461,
-0.936823075491869));
#57235=CARTESIAN_POINT('Ctrl Pts',(-0.063457605803671,-0.489180848883629,
-0.944695538311129));
#57236=CARTESIAN_POINT('Ctrl Pts',(-0.223806338772403,-0.468380061790797,
-0.952568001130388));
#57237=CARTESIAN_POINT('Ctrl Pts',(-0.372935857020711,-0.361092794313646,
-0.960440463949648));
#57238=CARTESIAN_POINT('Ctrl Pts',(-0.443631886793136,-0.215674568896387,
-0.968312926768907));
#57239=CARTESIAN_POINT('Ctrl Pts',(-0.475969230128613,-0.149158258182883,
-0.971913900315818));
#57240=CARTESIAN_POINT('Ctrl Pts',(-0.491896136050658,-0.0746639050419697,
-0.97551487386273));
#57241=CARTESIAN_POINT('Ctrl Pts',(-0.491746356789813,-0.00010883115493171,
-0.979115847409641));
#57242=CARTESIAN_POINT('Ctrl Pts',(-0.491736157223136,-8.20785977434006E-5,
-1.00088415259036));
#57243=CARTESIAN_POINT('Ctrl Pts',(-0.491851600629084,-0.0763714006472224,
-0.997199605606902));
#57244=CARTESIAN_POINT('Ctrl Pts',(-0.475143152162094,-0.152612842159027,
-0.993515058623445));
#57245=CARTESIAN_POINT('Ctrl Pts',(-0.441342370069444,-0.220321653526826,
-0.989830511639988));
#57246=CARTESIAN_POINT('Ctrl Pts',(-0.369123071067154,-0.36498939760024,
-0.981958048820729));
#57247=CARTESIAN_POINT('Ctrl Pts',(-0.218875066921732,-0.470704585739309,
-0.974085586001469));
#57248=CARTESIAN_POINT('Ctrl Pts',(-0.0583167449524224,-0.489820248550804,
-0.966213123182209));
#57249=CARTESIAN_POINT('Ctrl Pts',(0.102241577016886,-0.508935911362299,
-0.95834066036295));
#57250=CARTESIAN_POINT('Ctrl Pts',(0.273110216810081,-0.441452048846223,
-0.950468197543691));
#57251=CARTESIAN_POINT('Ctrl Pts',(0.377276845346877,-0.317784361800476,
-0.942595734724432));
#57252=CARTESIAN_POINT('Ctrl Pts',(0.481443473883674,-0.194116674754727,
-0.934723271905173));
#57253=CARTESIAN_POINT('Ctrl Pts',(0.518908091164071,-0.014265163179308,
-0.926850809085913));
#57254=CARTESIAN_POINT('Ctrl Pts',(0.472784992262523,0.140709167173152,
-0.918978346266654));
#57255=CARTESIAN_POINT('Ctrl Pts',(0.426661893360975,0.295683497525611,
-0.911105883447394));
#57256=CARTESIAN_POINT('Ctrl Pts',(0.296951078277482,0.425780646655112,
-0.903233420628134));
#57257=CARTESIAN_POINT('Ctrl Pts',(0.142114602924627,0.472364433749384,
-0.895360957808875));
#57258=CARTESIAN_POINT('Ctrl Pts',(-0.0127218724282286,0.518948220843657,
-0.887488494989616));
#57259=CARTESIAN_POINT('Ctrl Pts',(-0.192684008050446,0.482018645902701,
-0.879616032170357));
#57260=CARTESIAN_POINT('Ctrl Pts',(-0.316660938750639,0.378220264536789,
-0.871743569351098));
#57261=CARTESIAN_POINT('Ctrl Pts',(-0.426160194810032,0.286543164002481,
-0.864790430430852));
#57262=CARTESIAN_POINT('Ctrl Pts',(-0.491986368099344,0.142702872821624,
-0.857837291510605));
#57263=CARTESIAN_POINT('Ctrl Pts',(-0.493025735351581,-0.000302692969106977,
-0.850884152590359));
#57264=CARTESIAN_POINT('Origin',(0.,0.,-0.785));
#57265=CARTESIAN_POINT('',(-0.492442945015723,0.000430954536069797,-0.679115847409641));
#57266=CARTESIAN_POINT('',(-0.492493380507229,0.000430700144442887,-0.700884152590359));
#57267=CARTESIAN_POINT('',(-0.4925,-6.03138548580071E-17,-0.785));
#57268=CARTESIAN_POINT('Ctrl Pts',(-0.492442945015723,0.000430954536069797,
-0.679115847409641));
#57269=CARTESIAN_POINT('Ctrl Pts',(-0.492794956060319,0.0402362573843546,
-0.681045320031617));
#57270=CARTESIAN_POINT('Ctrl Pts',(-0.488365618774981,0.0799642458113595,
-0.682974792653592));
#57271=CARTESIAN_POINT('Ctrl Pts',(-0.478850766148977,0.118434430852565,
-0.684904265275568));
#57272=CARTESIAN_POINT('Ctrl Pts',(-0.440029109559597,0.27539706299233,
-0.692776728094828));
#57273=CARTESIAN_POINT('Ctrl Pts',(-0.316547316553595,0.411420655704654,
-0.700649190914088));
#57274=CARTESIAN_POINT('Ctrl Pts',(-0.164059955984402,0.465197916472846,
-0.708521653733347));
#57275=CARTESIAN_POINT('Ctrl Pts',(-0.0115725954152106,0.518975177241037,
-0.716394116552607));
#57276=CARTESIAN_POINT('Ctrl Pts',(0.16992033271717,0.490506106065098,-0.724266579371865));
#57277=CARTESIAN_POINT('Ctrl Pts',(0.298618018623332,0.392622018743623,
-0.732139042191125));
#57278=CARTESIAN_POINT('Ctrl Pts',(0.427315704529493,0.294737931422147,
-0.740011505010384));
#57279=CARTESIAN_POINT('Ctrl Pts',(0.503218148209435,0.127438827955136,
-0.747883967829644));
#57280=CARTESIAN_POINT('Ctrl Pts',(0.49211530399918,-0.0338717909113338,
-0.755756430648903));
#57281=CARTESIAN_POINT('Ctrl Pts',(0.481012459788925,-0.195182409777806,
-0.763628893468163));
#57282=CARTESIAN_POINT('Ctrl Pts',(0.382904327688472,-0.350504544043738,
-0.771501356287422));
#57283=CARTESIAN_POINT('Ctrl Pts',(0.242009295357658,-0.42983284147396,
-0.779373819106681));
#57284=CARTESIAN_POINT('Ctrl Pts',(0.101114263026846,-0.509161138904182,
-0.78724628192594));
#57285=CARTESIAN_POINT('Ctrl Pts',(-0.082567669534326,-0.512495599498696,
-0.7951187447452));
#57286=CARTESIAN_POINT('Ctrl Pts',(-0.22624908475085,-0.438333346094748,
-0.80299120756446));
#57287=CARTESIAN_POINT('Ctrl Pts',(-0.369930499967376,-0.364171092690799,
-0.810863670383719));
#57288=CARTESIAN_POINT('Ctrl Pts',(-0.473611397839254,-0.212512125288386,
-0.818736133202978));
#57289=CARTESIAN_POINT('Ctrl Pts',(-0.490561685389237,-0.0517107675186028,
-0.826608596022238));
#57290=CARTESIAN_POINT('Ctrl Pts',(-0.492361149036649,-0.0346398950093308,
-0.827444346484705));
#57291=CARTESIAN_POINT('Ctrl Pts',(-0.493183140477961,-0.0174659858392047,
-0.828280096947173));
#57292=CARTESIAN_POINT('Ctrl Pts',(-0.493065289251647,-0.000280683390702752,
-0.829115847409641));
#57293=CARTESIAN_POINT('Ctrl Pts',(-0.493025735351581,-0.000302692969106977,
-0.850884152590359));
#57294=CARTESIAN_POINT('Ctrl Pts',(-0.49316315748075,-0.0192104748833397,
-0.849964828691345));
#57295=CARTESIAN_POINT('Ctrl Pts',(-0.492168017944618,-0.0381036646601338,
-0.849045504792332));
#57296=CARTESIAN_POINT('Ctrl Pts',(-0.489991515851596,-0.056859766351132,
-0.848126180893318));
#57297=CARTESIAN_POINT('Ctrl Pts',(-0.471353436474192,-0.21747422808227,
-0.840253718074059));
#57298=CARTESIAN_POINT('Ctrl Pts',(-0.366085551941217,-0.368035963753677,
-0.8323812552548));
#57299=CARTESIAN_POINT('Ctrl Pts',(-0.221633227142547,-0.440685183847334,
-0.824508792435541));
#57300=CARTESIAN_POINT('Ctrl Pts',(-0.0771809023438781,-0.51333440394099,
-0.816636329616282));
#57301=CARTESIAN_POINT('Ctrl Pts',(0.106455862720485,-0.508071108456897,
-0.808763866797022));
#57302=CARTESIAN_POINT('Ctrl Pts',(0.246510007949834,-0.427267521134977,
-0.800891403977762));
#57303=CARTESIAN_POINT('Ctrl Pts',(0.386564153179185,-0.346463933813055,
-0.793018941158503));
#57304=CARTESIAN_POINT('Ctrl Pts',(0.483035678573522,-0.190120054653303,
-0.785146478339243));
#57305=CARTESIAN_POINT('Ctrl Pts',(0.492443832674891,-0.0287017472764125,
-0.777274015519984));
#57306=CARTESIAN_POINT('Ctrl Pts',(0.50185198677626,0.132716560100476,-0.769401552700724));
#57307=CARTESIAN_POINT('Ctrl Pts',(0.424196769584665,0.299209295694505,
-0.761529089881465));
#57308=CARTESIAN_POINT('Ctrl Pts',(0.294478220586881,0.395736397411412,
-0.753656627062206));
#57309=CARTESIAN_POINT('Ctrl Pts',(0.164759671589095,0.49226349912832,-0.745784164242946));
#57310=CARTESIAN_POINT('Ctrl Pts',(-0.0170222092148785,0.518824966968104,
-0.737911701423687));
#57311=CARTESIAN_POINT('Ctrl Pts',(-0.16893637796105,0.463449262419794,
-0.730039238604428));
#57312=CARTESIAN_POINT('Ctrl Pts',(-0.32085054670722,0.408073557871484,
-0.722166775785168));
#57313=CARTESIAN_POINT('Ctrl Pts',(-0.442897003395587,0.270760680935079,
-0.714294312965909));
#57314=CARTESIAN_POINT('Ctrl Pts',(-0.480068100660248,0.113399018360725,
-0.706421850146649));
#57315=CARTESIAN_POINT('Ctrl Pts',(-0.488783810056108,0.0765015732494849,
-0.704575950961219));
#57316=CARTESIAN_POINT('Ctrl Pts',(-0.492833179805818,0.0385018713240789,
-0.702730051775789));
#57317=CARTESIAN_POINT('Ctrl Pts',(-0.492493380507229,0.000430700144442887,
-0.700884152590359));
#57318=CARTESIAN_POINT('Origin',(0.,0.,-0.785));
#57319=CARTESIAN_POINT('',(-0.491840351485494,-0.000235604174339266,-0.529115847409641));
#57320=CARTESIAN_POINT('',(-0.491816277089331,-0.000212068874708314,-0.550884152590359));
#57321=CARTESIAN_POINT('',(-0.4925,-6.03138548580071E-17,-0.785));
#57322=CARTESIAN_POINT('Ctrl Pts',(-0.491840351485494,-0.000235604174339266,
-0.529115847409641));
#57323=CARTESIAN_POINT('Ctrl Pts',(-0.491412743741431,0.0969174984233381,
-0.53381054311606));
#57324=CARTESIAN_POINT('Ctrl Pts',(-0.463541921665293,0.194296900018551,
-0.53850523882248));
#57325=CARTESIAN_POINT('Ctrl Pts',(-0.40989902803581,0.274422225108048,
-0.543199934528899));
#57326=CARTESIAN_POINT('Ctrl Pts',(-0.319946087094793,0.408783146900192,
-0.551072397348158));
#57327=CARTESIAN_POINT('Ctrl Pts',(-0.157523578784168,0.494626608342158,
-0.558944860167418));
#57328=CARTESIAN_POINT('Ctrl Pts',(0.00416292928221056,0.493262040552515,
-0.566817322986677));
#57329=CARTESIAN_POINT('Ctrl Pts',(0.165849437348594,0.491897472762873,
-0.574689785805937));
#57330=CARTESIAN_POINT('Ctrl Pts',(0.326799945170732,0.403324875741616,
-0.582562248625196));
#57331=CARTESIAN_POINT('Ctrl Pts',(0.414472332492721,0.267464869118486,
-0.590434711444456));
#57332=CARTESIAN_POINT('Ctrl Pts',(0.502144719814708,0.13160486249536,-0.598307174263715));
#57333=CARTESIAN_POINT('Ctrl Pts',(0.516538986636549,-0.0515425537296376,
-0.606179637082975));
#57334=CARTESIAN_POINT('Ctrl Pts',(0.451167482309357,-0.199430874191682,
-0.614052099902234));
#57335=CARTESIAN_POINT('Ctrl Pts',(0.385795977982164,-0.347319194653728,
-0.621924562721493));
#57336=CARTESIAN_POINT('Ctrl Pts',(0.240658702505937,-0.459948419352821,
-0.629797025540753));
#57337=CARTESIAN_POINT('Ctrl Pts',(0.0811705830822261,-0.486555348430648,
-0.637669488360012));
#57338=CARTESIAN_POINT('Ctrl Pts',(-0.0783175363414848,-0.513162277508476,
-0.645541951179271));
#57339=CARTESIAN_POINT('Ctrl Pts',(-0.252156499712679,-0.453746910965039,
-0.653414413998531));
#57340=CARTESIAN_POINT('Ctrl Pts',(-0.361995221311897,-0.335088391909719,
-0.661286876817791));
#57341=CARTESIAN_POINT('Ctrl Pts',(-0.44491342121109,-0.245512050711285,
-0.667229867015074));
#57342=CARTESIAN_POINT('Ctrl Pts',(-0.491358711861264,-0.122173803848648,
-0.673172857212357));
#57343=CARTESIAN_POINT('Ctrl Pts',(-0.492442945015723,0.000430954536069797,
-0.679115847409641));
#57344=CARTESIAN_POINT('Ctrl Pts',(-0.492493380507229,0.000430700144442887,
-0.700884152590359));
#57345=CARTESIAN_POINT('Ctrl Pts',(-0.491383990508121,-0.123865543951382,
-0.69485758895653));
#57346=CARTESIAN_POINT('Ctrl Pts',(-0.443489685503747,-0.248923591237708,
-0.688831025322701));
#57347=CARTESIAN_POINT('Ctrl Pts',(-0.358456136920689,-0.338871533976663,
-0.682804461688872));
#57348=CARTESIAN_POINT('Ctrl Pts',(-0.247377338075509,-0.456369975527401,
-0.674931998869612));
#57349=CARTESIAN_POINT('Ctrl Pts',(-0.0729240025441891,-0.51395641041657,
-0.667059536050353));
#57350=CARTESIAN_POINT('Ctrl Pts',(0.086275879790834,-0.485676014645106,
-0.659187073231093));
#57351=CARTESIAN_POINT('Ctrl Pts',(0.245475762125855,-0.457395618873642,
-0.651314610411833));
#57352=CARTESIAN_POINT('Ctrl Pts',(0.38942219126458,-0.343248392441546,
-0.643442147592574));
#57353=CARTESIAN_POINT('Ctrl Pts',(0.453236967301004,-0.194681714887699,
-0.635569684773315));
#57354=CARTESIAN_POINT('Ctrl Pts',(0.517051743337429,-0.0461150373338516,
-0.627697221954055));
#57355=CARTESIAN_POINT('Ctrl Pts',(0.500734866271556,0.136871091341746,
-0.619824759134797));
#57356=CARTESIAN_POINT('Ctrl Pts',(0.411640527669831,0.271802859830283,
-0.611952296315537));
#57357=CARTESIAN_POINT('Ctrl Pts',(0.322546189068105,0.406734628318821,
-0.604079833496278));
#57358=CARTESIAN_POINT('Ctrl Pts',(0.160674388930523,0.493612036620296,
-0.596207370677018));
#57359=CARTESIAN_POINT('Ctrl Pts',(-0.00101751587672065,0.493278504794958,
-0.588334907857758));
#57360=CARTESIAN_POINT('Ctrl Pts',(-0.162709420683966,0.49294497296962,
-0.580462445038499));
#57361=CARTESIAN_POINT('Ctrl Pts',(-0.324221430160874,0.405400501017469,
-0.57258998221924));
#57362=CARTESIAN_POINT('Ctrl Pts',(-0.412758348824488,0.270102321606191,
-0.56471751939998));
#57363=CARTESIAN_POINT('Ctrl Pts',(-0.464616905254506,0.190854383257034,
-0.560106397130107));
#57364=CARTESIAN_POINT('Ctrl Pts',(-0.491439361299384,0.0952232297534331,
-0.555495274860233));
#57365=CARTESIAN_POINT('Ctrl Pts',(-0.491816277089331,-0.000212068874708314,
-0.550884152590359));
#57366=CARTESIAN_POINT('Origin',(0.,0.,-0.785));
#57367=CARTESIAN_POINT('',(-0.493221679829005,-0.00014905999630227,-0.379115847409641));
#57368=CARTESIAN_POINT('',(-0.493197442025473,-0.000177332146063924,-0.400884152590359));
#57369=CARTESIAN_POINT('',(-0.4925,-6.03138548580071E-17,-0.785));
#57370=CARTESIAN_POINT('Ctrl Pts',(-0.493221679829005,-0.00014905999630227,
-0.379115847409641));
#57371=CARTESIAN_POINT('Ctrl Pts',(-0.492603881529428,0.153118260426883,
-0.386575766200504));
#57372=CARTESIAN_POINT('Ctrl Pts',(-0.415450443578965,0.306923075433429,
-0.394035684991367));
#57373=CARTESIAN_POINT('Ctrl Pts',(-0.291948826220119,0.397606162425599,
-0.40149560378223));
#57374=CARTESIAN_POINT('Ctrl Pts',(-0.161617395271197,0.493304152001024,
-0.409368066601489));
#57375=CARTESIAN_POINT('Ctrl Pts',(0.0203301985725902,0.518705930657618,
-0.417240529420749));
#57376=CARTESIAN_POINT('Ctrl Pts',(0.171888191256297,0.462362651006137,
-0.425112992240008));
#57377=CARTESIAN_POINT('Ctrl Pts',(0.32344618394,0.406019371354658,-0.432985455059267));
#57378=CARTESIAN_POINT('Ctrl Pts',(0.444614575463624,0.267931033395105,
-0.440857917878527));
#57379=CARTESIAN_POINT('Ctrl Pts',(0.480781488250625,0.110335528963639,
-0.448730380697786));
#57380=CARTESIAN_POINT('Ctrl Pts',(0.516948401037627,-0.0472599754678293,
-0.456602843517046));
#57381=CARTESIAN_POINT('Ctrl Pts',(0.468113835088005,-0.224362646371213,
-0.464475306336305));
#57382=CARTESIAN_POINT('Ctrl Pts',(0.356288044656636,-0.341150408155024,
-0.472347769155565));
#57383=CARTESIAN_POINT('Ctrl Pts',(0.244462254225269,-0.457938169938832,
-0.480220231974824));
#57384=CARTESIAN_POINT('Ctrl Pts',(0.0696452393121575,-0.514411022603067,
-0.488092694794083));
#57385=CARTESIAN_POINT('Ctrl Pts',(-0.0893710915641801,-0.485116046552094,
-0.495965157613343));
#57386=CARTESIAN_POINT('Ctrl Pts',(-0.248387422440518,-0.45582107050112,
-0.503837620432602));
#57387=CARTESIAN_POINT('Ctrl Pts',(-0.391603069280081,-0.340758265734937,
-0.511710083251862));
#57388=CARTESIAN_POINT('Ctrl Pts',(-0.454469205914159,-0.191787672280683,
-0.519582546071121));
#57389=CARTESIAN_POINT('Ctrl Pts',(-0.479845501248111,-0.131654793469102,
-0.522760313183961));
#57390=CARTESIAN_POINT('Ctrl Pts',(-0.492129792572042,-0.0659970408363866,
-0.525938080296801));
#57391=CARTESIAN_POINT('Ctrl Pts',(-0.491840351485494,-0.000235604174339266,
-0.529115847409641));
#57392=CARTESIAN_POINT('Ctrl Pts',(-0.491816277089331,-0.000212068874708314,
-0.550884152590359));
#57393=CARTESIAN_POINT('Ctrl Pts',(-0.492082860944087,-0.06771125693402,
-0.547622812040973));
#57394=CARTESIAN_POINT('Ctrl Pts',(-0.479120309212638,-0.135112470413207,
-0.544361471491588));
#57395=CARTESIAN_POINT('Ctrl Pts',(-0.452429949774634,-0.196549889717956,
-0.541100130942202));
#57396=CARTESIAN_POINT('Ctrl Pts',(-0.388002804210847,-0.344852034760429,
-0.533227668122942));
#57397=CARTESIAN_POINT('Ctrl Pts',(-0.243586685232952,-0.458404437974975,
-0.525355205303683));
#57398=CARTESIAN_POINT('Ctrl Pts',(-0.0842714866745568,-0.486027813145279,
-0.517482742484424));
#57399=CARTESIAN_POINT('Ctrl Pts',(0.0750437118838385,-0.513651188315582,
-0.509610279665164));
#57400=CARTESIAN_POINT('Ctrl Pts',(0.249257990022733,-0.455345535441644,
-0.501737816845905));
#57401=CARTESIAN_POINT('Ctrl Pts',(0.35985110298877,-0.337389837552566,
-0.493865354026646));
#57402=CARTESIAN_POINT('Ctrl Pts',(0.470444215954808,-0.219434139663487,
-0.485992891207386));
#57403=CARTESIAN_POINT('Ctrl Pts',(0.517416163747986,-0.0418283967592656,
-0.478120428388126));
#57404=CARTESIAN_POINT('Ctrl Pts',(0.479596186721551,0.115378576999044,
-0.470247965568867));
#57405=CARTESIAN_POINT('Ctrl Pts',(0.441776209695117,0.272585550757351,
-0.462375502749608));
#57406=CARTESIAN_POINT('Ctrl Pts',(0.319164307849076,0.409393755369748,
-0.454503039930348));
#57407=CARTESIAN_POINT('Ctrl Pts',(0.167022978541554,0.464142266181422,
-0.446630577111089));
#57408=CARTESIAN_POINT('Ctrl Pts',(0.0148816492340293,0.518890776993097,
-0.43875811429183));
#57409=CARTESIAN_POINT('Ctrl Pts',(-0.166789107534976,0.491579594004046,
-0.43088565147257));
#57410=CARTESIAN_POINT('Ctrl Pts',(-0.296108328455227,0.394518158722321,
-0.423013188653311));
#57411=CARTESIAN_POINT('Ctrl Pts',(-0.417277936538399,0.303573471696024,
-0.415636843298994));
#57412=CARTESIAN_POINT('Ctrl Pts',(-0.492486417081148,0.151392754252931,
-0.408260497944676));
#57413=CARTESIAN_POINT('Ctrl Pts',(-0.493197442025473,-0.000177332146063924,
-0.400884152590359));
#57414=CARTESIAN_POINT('Origin',(0.,0.,-0.785));
#57415=CARTESIAN_POINT('',(-0.492199160006355,0.000404087486738508,-0.229115847409641));
#57416=CARTESIAN_POINT('',(-0.492244893268066,0.000412969905903395,-0.250884152590359));
#57417=CARTESIAN_POINT('',(-0.4925,-6.03138548580071E-17,-0.785));
#57418=CARTESIAN_POINT('Ctrl Pts',(-0.492199160006355,0.000404087486738508,
-0.229115847409641));
#57419=CARTESIAN_POINT('Ctrl Pts',(-0.492584826275126,0.0490014356714362,
-0.231468526465688));
#57420=CARTESIAN_POINT('Ctrl Pts',(-0.485956433324197,0.0974958164498649,
-0.233821205521735));
#57421=CARTESIAN_POINT('Ctrl Pts',(-0.471877297107457,0.143720885963992,
-0.236173884577782));
#57422=CARTESIAN_POINT('Ctrl Pts',(-0.424766121399625,0.298397802108716,
-0.244046347397041));
#57423=CARTESIAN_POINT('Ctrl Pts',(-0.294230090276064,0.427665580216661,
-0.251918810216301));
#57424=CARTESIAN_POINT('Ctrl Pts',(-0.139100117626822,0.473261186203299,
-0.259791273035561));
#57425=CARTESIAN_POINT('Ctrl Pts',(0.0160298550224196,0.518856792189937,
-0.26766373585482));
#57426=CARTESIAN_POINT('Ctrl Pts',(0.195753769197341,0.480780226055272,
-0.275536198674079));
#57427=CARTESIAN_POINT('Ctrl Pts',(0.319066529828403,0.376193347566822,
-0.283408661493339));
#57428=CARTESIAN_POINT('Ctrl Pts',(0.442379290459466,0.271606469078371,
-0.291281124312598));
#57429=CARTESIAN_POINT('Ctrl Pts',(0.509280897546665,0.100509278236134,
-0.299153587131858));
#57430=CARTESIAN_POINT('Ctrl Pts',(0.489618910158042,-0.0599830637448122,
-0.307026049951117));
#57431=CARTESIAN_POINT('Ctrl Pts',(0.469956922769419,-0.220475405725756,
-0.314898512770376));
#57432=CARTESIAN_POINT('Ctrl Pts',(0.363731340904977,-0.37036289884541,
-0.322770975589636));
#57433=CARTESIAN_POINT('Ctrl Pts',(0.218818741885396,-0.442089549274763,
-0.330643438408895));
#57434=CARTESIAN_POINT('Ctrl Pts',(0.0739061428658151,-0.513816199704116,
-0.338515901228154));
#57435=CARTESIAN_POINT('Ctrl Pts',(-0.109693473308903,-0.507382007443169,
-0.346388364047414));
#57436=CARTESIAN_POINT('Ctrl Pts',(-0.24922956536185,-0.425686980138714,
-0.354260826866673));
#57437=CARTESIAN_POINT('Ctrl Pts',(-0.388765657414798,-0.34399195283426,
-0.362133289685933));
#57438=CARTESIAN_POINT('Ctrl Pts',(-0.484238225345974,-0.187036090486295,
-0.370005752505192));
#57439=CARTESIAN_POINT('Ctrl Pts',(-0.492616875284533,-0.025561059065186,
-0.377878215324452));
#57440=CARTESIAN_POINT('Ctrl Pts',(-0.493055945252538,-0.0170992140902034,
-0.378290759352848));
#57441=CARTESIAN_POINT('Ctrl Pts',(-0.493255844946132,-0.00862495893857167,
-0.378703303381244));
#57442=CARTESIAN_POINT('Ctrl Pts',(-0.493221679829005,-0.00014905999630227,
-0.379115847409641));
#57443=CARTESIAN_POINT('Ctrl Pts',(-0.493197442025473,-0.000177332146063924,
-0.400884152590359));
#57444=CARTESIAN_POINT('Ctrl Pts',(-0.493245264066869,-0.0103716171765687,
-0.400388035125417));
#57445=CARTESIAN_POINT('Ctrl Pts',(-0.492956087592501,-0.0205631399415184,
-0.399891917660475));
#57446=CARTESIAN_POINT('Ctrl Pts',(-0.492321230439843,-0.0307330836272979,
-0.399395800195532));
#57447=CARTESIAN_POINT('Ctrl Pts',(-0.482247226432713,-0.19211120312079,
-0.391523337376273));
#57448=CARTESIAN_POINT('Ctrl Pts',(-0.385131533346962,-0.348055754533375,
-0.383650874557014));
#57449=CARTESIAN_POINT('Ctrl Pts',(-0.244745220248979,-0.428280861698101,
-0.375778411737754));
#57450=CARTESIAN_POINT('Ctrl Pts',(-0.104358907150996,-0.508505968862826,
-0.367905948918495));
#57451=CARTESIAN_POINT('Ctrl Pts',(0.0792980259592206,-0.51301163177969,
-0.360033486099235));
#57452=CARTESIAN_POINT('Ctrl Pts',(0.223449398871474,-0.439767088000122,
-0.352161023279976));
#57453=CARTESIAN_POINT('Ctrl Pts',(0.367600771783729,-0.366522544220555,
-0.344288560460717));
#57454=CARTESIAN_POINT('Ctrl Pts',(0.472246584498022,-0.215527793744555,
-0.336416097641457));
#57455=CARTESIAN_POINT('Ctrl Pts',(0.49022190455631,-0.0548378132669632,
-0.328543634822198));
#57456=CARTESIAN_POINT('Ctrl Pts',(0.508197224614599,0.105852167210629,
-0.320671172002939));
#57457=CARTESIAN_POINT('Ctrl Pts',(0.439502052016882,0.276237377689811,
-0.312798709183679));
#57458=CARTESIAN_POINT('Ctrl Pts',(0.315097926507763,0.379523419652241,
-0.30492624636442));
#57459=CARTESIAN_POINT('Ctrl Pts',(0.190693800998646,0.482809461614669,
-0.297053783545161));
#57460=CARTESIAN_POINT('Ctrl Pts',(0.0105807225781267,0.518996335060344,
-0.289181320725901));
#57461=CARTESIAN_POINT('Ctrl Pts',(-0.144062197569475,0.471774143744356,
-0.281308857906642));
#57462=CARTESIAN_POINT('Ctrl Pts',(-0.298705117717077,0.424551952428368,
-0.273436395087382));
#57463=CARTESIAN_POINT('Ctrl Pts',(-0.427877879591762,0.293920696350717,
-0.265563932268123));
#57464=CARTESIAN_POINT('Ctrl Pts',(-0.473361346043439,0.138757445912334,
-0.257691469448863));
#57465=CARTESIAN_POINT('Ctrl Pts',(-0.486471193836867,0.0940342364678234,
-0.255422363829362));
#57466=CARTESIAN_POINT('Ctrl Pts',(-0.492628267870041,0.0472729478900636,
-0.25315325820986));
#57467=CARTESIAN_POINT('Ctrl Pts',(-0.492244893268066,0.000412969905903395,
-0.250884152590359));
#57468=CARTESIAN_POINT('Origin',(0.,0.,-0.785));
#57469=CARTESIAN_POINT('',(-0.492093596265288,-0.000318355522334279,-0.0791158474096402));
#57470=CARTESIAN_POINT('',(-0.491975623968706,-0.000315807630563663,-0.100884152590359));
#57471=CARTESIAN_POINT('',(-0.4925,-6.03138548580071E-17,-0.785));
#57472=CARTESIAN_POINT('Ctrl Pts',(-0.492093596265288,-0.000318355522334279,
-0.0791158474096402));
#57473=CARTESIAN_POINT('Ctrl Pts',(-0.491378781731003,0.105499822008811,
-0.0842337495501311));
#57474=CARTESIAN_POINT('Ctrl Pts',(-0.457753103959109,0.211702860821235,
-0.089351651690622));
#57475=CARTESIAN_POINT('Ctrl Pts',(-0.394687347650209,0.295813436971342,
-0.0944695538311129));
#57476=CARTESIAN_POINT('Ctrl Pts',(-0.297678298223042,0.425194063109043,
-0.102342016650372));
#57477=CARTESIAN_POINT('Ctrl Pts',(-0.131010407576646,0.502301209513945,
-0.110214479469632));
#57478=CARTESIAN_POINT('Ctrl Pts',(0.0303537882400381,0.49234839688357,
-0.118086942288891));
#57479=CARTESIAN_POINT('Ctrl Pts',(0.191717984056725,0.482395584253196,
-0.12595940510815));
#57480=CARTESIAN_POINT('Ctrl Pts',(0.347778485043697,0.385382812587542,
-0.13383186792741));
#57481=CARTESIAN_POINT('Ctrl Pts',(0.428116051422676,0.245052162104028,
-0.141704330746669));
#57482=CARTESIAN_POINT('Ctrl Pts',(0.508453617801651,0.104721511620518,
-0.149576793565929));
#57483=CARTESIAN_POINT('Ctrl Pts',(0.513068249572635,-0.0789270176808498,
-0.157449256385188));
#57484=CARTESIAN_POINT('Ctrl Pts',(0.43992221351322,-0.223130098498712,
-0.165321719204447));
#57485=CARTESIAN_POINT('Ctrl Pts',(0.366776177453803,-0.36733317931658,
-0.173194182023707));
#57486=CARTESIAN_POINT('Ctrl Pts',(0.215869473563981,-0.472090811650941,
-0.181066644842966));
#57487=CARTESIAN_POINT('Ctrl Pts',(0.0551954744401251,-0.490182910244527,
-0.188939107662226));
#57488=CARTESIAN_POINT('Ctrl Pts',(-0.105478524683729,-0.508275008838114,
-0.196811570481485));
#57489=CARTESIAN_POINT('Ctrl Pts',(-0.275919819041619,-0.439701573690924,
-0.204684033300745));
#57490=CARTESIAN_POINT('Ctrl Pts',(-0.379297306074508,-0.315371829026578,
-0.212556496120004));
#57491=CARTESIAN_POINT('Ctrl Pts',(-0.451780515904327,-0.228197926572105,
-0.218076279883216));
#57492=CARTESIAN_POINT('Ctrl Pts',(-0.491294321582725,-0.113613526924198,
-0.223596063646428));
#57493=CARTESIAN_POINT('Ctrl Pts',(-0.492199160006355,0.000404087486738508,
-0.229115847409641));
#57494=CARTESIAN_POINT('Ctrl Pts',(-0.492244893268066,0.000412969905903395,
-0.250884152590359));
#57495=CARTESIAN_POINT('Ctrl Pts',(-0.491298183331906,-0.115303633482406,
-0.245280795390601));
#57496=CARTESIAN_POINT('Ctrl Pts',(-0.450467838346037,-0.231622044558184,
-0.239677438190843));
#57497=CARTESIAN_POINT('Ctrl Pts',(-0.375962843028185,-0.319338025106157,
-0.234074080991085));
#57498=CARTESIAN_POINT('Ctrl Pts',(-0.271286702532588,-0.442575000887142,
-0.226201618171826));
#57499=CARTESIAN_POINT('Ctrl Pts',(-0.100140250512727,-0.509353707650003,
-0.218329155352567));
#57500=CARTESIAN_POINT('Ctrl Pts',(0.0603374458436118,-0.489575667285348,
-0.210456692533307));
#57501=CARTESIAN_POINT('Ctrl Pts',(0.220815142199958,-0.469797626920692,
-0.202584229714048));
#57502=CARTESIAN_POINT('Ctrl Pts',(0.370624082892782,-0.363462839428512,
-0.194711766894788));
#57503=CARTESIAN_POINT('Ctrl Pts',(0.442246704181642,-0.218498685373315,
-0.186839304075529));
#57504=CARTESIAN_POINT('Ctrl Pts',(0.513869325470499,-0.0735345313181219,
-0.178966841256269));
#57505=CARTESIAN_POINT('Ctrl Pts',(0.507305627355399,0.110058989300087,
-0.17109437843701));
#57506=CARTESIAN_POINT('Ctrl Pts',(0.425508298637621,0.249536520685491,
-0.163221915617751));
#57507=CARTESIAN_POINT('Ctrl Pts',(0.343710969919843,0.389014052070895,
-0.155349452798491));
#57508=CARTESIAN_POINT('Ctrl Pts',(0.186680010599389,0.484375594223496,
-0.147476989979232));
#57509=CARTESIAN_POINT('Ctrl Pts',(0.0252018055069099,0.492636420199208,
-0.139604527159972));
#57510=CARTESIAN_POINT('Ctrl Pts',(-0.136276399585572,0.50089724617492,
-0.131732064340713));
#57511=CARTESIAN_POINT('Ctrl Pts',(-0.302201850450079,0.422057355973741,
-0.123859601521453));
#57512=CARTESIAN_POINT('Ctrl Pts',(-0.39781102594903,0.291658920200447,
-0.115987138702194));
#57513=CARTESIAN_POINT('Ctrl Pts',(-0.458951742345601,0.20827096356799,
-0.110952809998249));
#57514=CARTESIAN_POINT('Ctrl Pts',(-0.491337168305235,0.103798543278651,
-0.105918481294304));
#57515=CARTESIAN_POINT('Ctrl Pts',(-0.491975623968706,-0.000315807630563663,
-0.100884152590359));
#57516=CARTESIAN_POINT('Origin',(0.,0.,-1.90478126690739));
#57517=CARTESIAN_POINT('',(-0.406714108344742,-0.000263120031215911,-0.0297812669073861));
#57518=CARTESIAN_POINT('',(-0.40704949043302,-3.9445486058054E-7,-0.000218733092610173));
#57519=CARTESIAN_POINT('',(-0.40705,-2.29167262861955E-14,-1.90478126690739));
#57520=CARTESIAN_POINT('',(-0.1293270056281,-0.385958842514677,0.));
#57521=CARTESIAN_POINT('Ctrl Pts',(-0.406714108344742,-0.000263120031215928,
-0.0297812669073861));
#57522=CARTESIAN_POINT('Ctrl Pts',(-0.407032085020554,-0.0473350676737868,
-0.0270267062286178));
#57523=CARTESIAN_POINT('Ctrl Pts',(-0.379781121781836,-0.216644350034151,
-0.0170996172594891));
#57524=CARTESIAN_POINT('Ctrl Pts',(-0.244382435473693,-0.347137952462494,
-0.00717252829036035));
#57525=CARTESIAN_POINT('Ctrl Pts',(-0.129150719006634,-0.38654594480115,
-6.28837260041593E-18));
#57526=CARTESIAN_POINT('',(-0.407032914766026,-0.00372944996920639,-2.22044604925031E-16));
#57527=CARTESIAN_POINT('Origin',(0.,0.,0.));
#57528=CARTESIAN_POINT('Ctrl Pts',(-0.40704949043302,-3.9445486056883E-7,
-0.000218733092610175));
#57529=CARTESIAN_POINT('Ctrl Pts',(-0.407049825054718,-0.00124330109335373,
-0.000145822061740043));
#57530=CARTESIAN_POINT('Ctrl Pts',(-0.407044304842328,-0.00248633476599664,
-7.29110308699103E-5));
#57531=CARTESIAN_POINT('Ctrl Pts',(-0.407032914766026,-0.00372944996921217,
2.22044604925031E-16));
#57532=CARTESIAN_POINT('Origin',(0.,0.,-1.90478126690739));
#57533=CARTESIAN_POINT('',(-0.406801356508805,0.000333977282159546,-0.179781266907386));
#57534=CARTESIAN_POINT('',(-0.406616604541039,-0.000261014205145876,-0.150218733092611));
#57535=CARTESIAN_POINT('',(-0.40705,-2.29167262861955E-14,-1.90478126690739));
#57536=CARTESIAN_POINT('Ctrl Pts',(-0.406801356508805,0.000333977282159493,
-0.179781266907386));
#57537=CARTESIAN_POINT('Ctrl Pts',(-0.406053509848213,-0.0939012916436638,
-0.174261483144174));
#57538=CARTESIAN_POINT('Ctrl Pts',(-0.32681765341167,-0.323673971963636,
-0.160869236561703));
#57539=CARTESIAN_POINT('Ctrl Pts',(0.053691564255565,-0.476763774871506,
-0.139604527159972));
#57540=CARTESIAN_POINT('Ctrl Pts',(0.427863587514561,-0.217018023145409,
-0.115987138702194));
#57541=CARTESIAN_POINT('Ctrl Pts',(0.416421643175193,0.238337106918288,
-0.0923697502444159));
#57542=CARTESIAN_POINT('Ctrl Pts',(0.0294708192559207,0.478879535587345,
-0.0687523617866379));
#57543=CARTESIAN_POINT('Ctrl Pts',(-0.335582261652634,0.309991567748977,
-0.0478895340076277));
#57544=CARTESIAN_POINT('Ctrl Pts',(-0.406123315946409,0.0871953351242249,
-0.0348991690478773));
#57545=CARTESIAN_POINT('Ctrl Pts',(-0.406714108344742,-0.000263120031215928,
-0.0297812669073861));
#57546=CARTESIAN_POINT('Ctrl Pts',(-0.406616604541039,-0.000261014205145928,
-0.150218733092611));
#57547=CARTESIAN_POINT('Ctrl Pts',(-0.406914088541965,-0.0487723759716419,
-0.147380598977297));
#57548=CARTESIAN_POINT('Ctrl Pts',(-0.376565976179168,-0.231490392209914,
-0.136670002042723));
#57549=CARTESIAN_POINT('Ctrl Pts',(-0.106905499254799,-0.467723490470255,
-0.118086942288891));
#57550=CARTESIAN_POINT('Ctrl Pts',(0.331923550485991,-0.346239581300314,
-0.0944695538311125));
#57551=CARTESIAN_POINT('Ctrl Pts',(0.472036117814807,0.0871616494771883,
-0.0708521653733347));
#57552=CARTESIAN_POINT('Ctrl Pts',(0.18569067875618,0.442363687480316,-0.0472347769155563));
#57553=CARTESIAN_POINT('Ctrl Pts',(-0.190742685458467,0.405446943649056,
-0.0275536198674078));
#57554=CARTESIAN_POINT('Ctrl Pts',(-0.37380969085203,0.198095302065577,
-0.0118816052597593));
#57555=CARTESIAN_POINT('Ctrl Pts',(-0.407031759908428,0.0658572197920024,
-0.00408205347136984));
#57556=CARTESIAN_POINT('Ctrl Pts',(-0.40704949043302,-3.9445486056883E-7,
-0.000218733092610175));
#57557=CARTESIAN_POINT('Origin',(0.,0.,-1.90478126690739));
#57558=CARTESIAN_POINT('',(-0.407646466546998,-0.000123197708628549,-0.329781266907387));
#57559=CARTESIAN_POINT('',(-0.406839154933536,0.000341318579049288,-0.300218733092611));
#57560=CARTESIAN_POINT('',(-0.40705,-2.29167262861955E-14,-1.90478126690739));
#57561=CARTESIAN_POINT('Ctrl Pts',(-0.407646466546998,-0.000123197708628555,
-0.329781266907387));
#57562=CARTESIAN_POINT('Ctrl Pts',(-0.407674703929589,-0.00712850667197845,
-0.329368722878991));
#57563=CARTESIAN_POINT('Ctrl Pts',(-0.404356705170022,-0.147786891764727,
-0.321083716031335));
#57564=CARTESIAN_POINT('Ctrl Pts',(-0.242405994059508,-0.414032097806954,
-0.30492624636442));
#57565=CARTESIAN_POINT('Ctrl Pts',(0.21282785627909,-0.429985628526655,
-0.281308857906642));
#57566=CARTESIAN_POINT('Ctrl Pts',(0.476213377687744,-0.0583407306117992,
-0.257691469448864));
#57567=CARTESIAN_POINT('Ctrl Pts',(0.310331352318132,0.365893451311033,
-0.234074080991085));
#57568=CARTESIAN_POINT('Ctrl Pts',(-0.135292724422396,0.460304007118841,
-0.210456692533307));
#57569=CARTESIAN_POINT('Ctrl Pts',(-0.383310271424921,0.214696131983949,
-0.192359087838741));
#57570=CARTESIAN_POINT('Ctrl Pts',(-0.407120108701099,0.0404995622132968,
-0.182133945963434));
#57571=CARTESIAN_POINT('Ctrl Pts',(-0.406801356508805,0.000333977282159493,
-0.179781266907386));
#57572=CARTESIAN_POINT('Ctrl Pts',(-0.406839154933536,0.000341318579049298,
-0.300218733092611));
#57573=CARTESIAN_POINT('Ctrl Pts',(-0.406056701574109,-0.0952981604244157,
-0.294615375892853));
#57574=CARTESIAN_POINT('Ctrl Pts',(-0.324898677082925,-0.326502977776057,
-0.281139555873836));
#57575=CARTESIAN_POINT('Ctrl Pts',(0.0586864453268738,-0.476171978247222,
-0.259791273035561));
#57576=CARTESIAN_POINT('Ctrl Pts',(0.430136573097502,-0.212515682316106,
-0.236173884577782));
#57577=CARTESIAN_POINT('Ctrl Pts',(0.413861933598501,0.242703054136536,
-0.212556496120004));
#57578=CARTESIAN_POINT('Ctrl Pts',(0.0245048656306335,0.479151271800793,
-0.188939107662225));
#57579=CARTESIAN_POINT('Ctrl Pts',(-0.337466212584372,0.30715981471096,
-0.168159853319762));
#57580=CARTESIAN_POINT('Ctrl Pts',(-0.406088922555631,0.0857892325717066,
-0.155253061796556));
#57581=CARTESIAN_POINT('Ctrl Pts',(-0.406616604541039,-0.000261014205145928,
-0.150218733092611));
#57582=CARTESIAN_POINT('Origin',(0.,0.,-1.90478126690739));
#57583=CARTESIAN_POINT('',(-0.406504802176995,-0.000194726252129646,-0.479781266907387));
#57584=CARTESIAN_POINT('',(-0.407626434063896,-0.000146564568675844,-0.450218733092611));
#57585=CARTESIAN_POINT('',(-0.40705,-2.29167262861955E-14,-1.90478126690739));
#57586=CARTESIAN_POINT('Ctrl Pts',(-0.406504802176995,-0.000194726252129608,
-0.479781266907387));
#57587=CARTESIAN_POINT('Ctrl Pts',(-0.406744024500403,-0.0545463867461071,
-0.476603499794547));
#57588=CARTESIAN_POINT('Ctrl Pts',(-0.371438645317141,-0.243248509798392,
-0.465553269862447));
#57589=CARTESIAN_POINT('Ctrl Pts',(-0.0869242056007438,-0.471834073964581,
-0.446630577111089));
#57590=CARTESIAN_POINT('Ctrl Pts',(0.346533251782296,-0.331810065779944,
-0.423013188653311));
#57591=CARTESIAN_POINT('Ctrl Pts',(0.467618186217581,0.1073146582275,-0.399395800195533));
#57592=CARTESIAN_POINT('Ctrl Pts',(0.167182082036718,0.449703640764164,
-0.375778411737755));
#57593=CARTESIAN_POINT('Ctrl Pts',(-0.276075204840169,0.387820308034648,
-0.352573567308372));
#57594=CARTESIAN_POINT('Ctrl Pts',(-0.407135857820417,0.126551853617785,
-0.33724118569825));
#57595=CARTESIAN_POINT('Ctrl Pts',(-0.407646466546998,-0.000123197708628555,
-0.329781266907387));
#57596=CARTESIAN_POINT('Ctrl Pts',(-0.407626434063896,-0.000146564568675865,
-0.450218733092611));
#57597=CARTESIAN_POINT('Ctrl Pts',(-0.407665958859733,-0.00857211527255664,
-0.449722615627669));
#57598=CARTESIAN_POINT('Ctrl Pts',(-0.403634411612907,-0.150656998330975,
-0.441354035343468));
#57599=CARTESIAN_POINT('Ctrl Pts',(-0.238044360971215,-0.416554973675746,
-0.425112992240007));
#57600=CARTESIAN_POINT('Ctrl Pts',(0.217331606272519,-0.427726730571028,
-0.40149560378223));
#57601=CARTESIAN_POINT('Ctrl Pts',(0.476800102102078,-0.0533363964720061,
-0.377878215324451));
#57602=CARTESIAN_POINT('Ctrl Pts',(0.306470944705725,0.369132435561808,
-0.354260826866673));
#57603=CARTESIAN_POINT('Ctrl Pts',(-0.140118061818574,0.458857512735786,
-0.330643438408895));
#57604=CARTESIAN_POINT('Ctrl Pts',(-0.38441204095114,0.211805201682357,
-0.312629407150874));
#57605=CARTESIAN_POINT('Ctrl Pts',(-0.407156013069039,0.039070971449013,
-0.302487838712113));
#57606=CARTESIAN_POINT('Ctrl Pts',(-0.406839154933536,0.000341318579049298,
-0.300218733092611));
#57607=CARTESIAN_POINT('Origin',(0.,0.,-1.90478126690739));
#57608=CARTESIAN_POINT('',(-0.407002844200305,0.000356182830250053,-0.629781266907387));
#57609=CARTESIAN_POINT('',(-0.406484904749669,-0.000175274386724683,-0.600218733092611));
#57610=CARTESIAN_POINT('',(-0.40705,-2.29167262861955E-14,-1.90478126690739));
#57611=CARTESIAN_POINT('Ctrl Pts',(-0.407002844200305,0.000356182830250049,
-0.629781266907387));
#57612=CARTESIAN_POINT('Ctrl Pts',(-0.406106728250001,-0.100976338795125,
-0.623838276710104));
#57613=CARTESIAN_POINT('Ctrl Pts',(-0.316870064410776,-0.337949636189232,
-0.61002282369356));
#57614=CARTESIAN_POINT('Ctrl Pts',(0.0789482169998913,-0.473233969566154,
-0.588334907857759));
#57615=CARTESIAN_POINT('Ctrl Pts',(0.438814986437033,-0.193970664507679,
-0.56471751939998));
#57616=CARTESIAN_POINT('Ctrl Pts',(0.40312451145329,0.260141959498729,-0.541100130942203));
#57617=CARTESIAN_POINT('Ctrl Pts',(0.00404895281978514,0.479757039402292,
-0.517482742484423));
#57618=CARTESIAN_POINT('Ctrl Pts',(-0.344488911026044,0.295547984959571,
-0.497043121139486));
#57619=CARTESIAN_POINT('Ctrl Pts',(-0.40615138546183,0.0801020664633769,
-0.484475962613807));
#57620=CARTESIAN_POINT('Ctrl Pts',(-0.406504802176995,-0.000194726252129608,
-0.479781266907387));
#57621=CARTESIAN_POINT('Ctrl Pts',(-0.406484904749669,-0.000175274386724725,
-0.600218733092611));
#57622=CARTESIAN_POINT('Ctrl Pts',(-0.406705235629013,-0.0559631820000021,
-0.596957392543226));
#57623=CARTESIAN_POINT('Ctrl Pts',(-0.370130649226088,-0.246139588399615,
-0.585823589174581));
#57624=CARTESIAN_POINT('Ctrl Pts',(-0.0819642213078552,-0.472720877576032,
-0.566817322986677));
#57625=CARTESIAN_POINT('Ctrl Pts',(0.349998754832881,-0.328152455226764,
-0.543199934528899));
#57626=CARTESIAN_POINT('Ctrl Pts',(0.466465341731633,0.112219631976251,
-0.51958254607112));
#57627=CARTESIAN_POINT('Ctrl Pts',(0.162450064697528,0.451434533625857,
-0.495965157613343));
#57628=CARTESIAN_POINT('Ctrl Pts',(-0.278538812073554,0.385139175342376,
-0.472843886620505));
#57629=CARTESIAN_POINT('Ctrl Pts',(-0.407038773752055,0.125125727144453,
-0.457595078446929));
#57630=CARTESIAN_POINT('Ctrl Pts',(-0.407626434063896,-0.000146564568675865,
-0.450218733092611));
#57631=CARTESIAN_POINT('Origin',(0.,0.,-1.90478126690739));
#57632=CARTESIAN_POINT('',(-0.407517210131742,-0.000231984110039767,-0.779781266907388));
#57633=CARTESIAN_POINT('',(-0.407044529006025,0.000355972576201596,-0.750218733092611));
#57634=CARTESIAN_POINT('',(-0.40705,-2.29167262861955E-14,-1.90478126690739));
#57635=CARTESIAN_POINT('Ctrl Pts',(-0.407517210131742,-0.000231984110039793,
-0.779781266907388));
#57636=CARTESIAN_POINT('Ctrl Pts',(-0.407614613871175,-0.0144355929662029,
-0.77894551644492));
#57637=CARTESIAN_POINT('Ctrl Pts',(-0.400535787639923,-0.16233387099766,
-0.770237303163193));
#57638=CARTESIAN_POINT('Ctrl Pts',(-0.220054620371515,-0.42633223545369,
-0.753656627062206));
#57639=CARTESIAN_POINT('Ctrl Pts',(0.235383332820519,-0.418064465798881,
-0.730039238604428));
#57640=CARTESIAN_POINT('Ctrl Pts',(0.478641699347353,-0.0329444165423497,
-0.70642185014665));
#57641=CARTESIAN_POINT('Ctrl Pts',(0.290442168180321,0.381872436653063,
-0.682804461688872));
#57642=CARTESIAN_POINT('Ctrl Pts',(-0.159568165198072,0.452461281864222,
-0.659187073231093));
#57643=CARTESIAN_POINT('Ctrl Pts',(-0.388696326414372,0.200061029798759,
-0.641512674970599));
#57644=CARTESIAN_POINT('Ctrl Pts',(-0.407293780435236,0.0332551646056748,
-0.631710739529363));
#57645=CARTESIAN_POINT('Ctrl Pts',(-0.407002844200305,0.000356182830250049,
-0.629781266907387));
#57646=CARTESIAN_POINT('Ctrl Pts',(-0.407044529006025,0.000355972576201576,
-0.750218733092611));
#57647=CARTESIAN_POINT('Ctrl Pts',(-0.406127620987465,-0.102374557696288,
-0.744192169458782));
#57648=CARTESIAN_POINT('Ctrl Pts',(-0.314834083697359,-0.340753452688454,
-0.730293143005694));
#57649=CARTESIAN_POINT('Ctrl Pts',(0.0839137360252065,-0.472378711028833,
-0.708521653733346));
#57650=CARTESIAN_POINT('Ctrl Pts',(0.440827811035869,-0.189351532231765,
-0.684904265275568));
#57651=CARTESIAN_POINT('Ctrl Pts',(0.400370238591211,0.264361180523987,
-0.66128687681779));
#57652=CARTESIAN_POINT('Ctrl Pts',(-0.000989657323522311,0.479773052904378,
-0.637669488360011));
#57653=CARTESIAN_POINT('Ctrl Pts',(-0.346156596104652,0.292681966063216,
-0.617313440451619));
#57654=CARTESIAN_POINT('Ctrl Pts',(-0.406173384805922,0.0787017577078716,
-0.604829855362485));
#57655=CARTESIAN_POINT('Ctrl Pts',(-0.406484904749669,-0.000175274386724725,
-0.600218733092611));
#57656=CARTESIAN_POINT('Origin',(0.,0.,-1.90478126690739));
#57657=CARTESIAN_POINT('',(-0.406427115799581,-8.9948673345385E-5,-0.929781266907387));
#57658=CARTESIAN_POINT('',(-0.407484518933728,-0.00025017497073776,-0.900218733092611));
#57659=CARTESIAN_POINT('',(-0.40705,-2.29167262861955E-14,-1.90478126690739));
#57660=CARTESIAN_POINT('Ctrl Pts',(-0.406427115799581,-8.99486733453581E-5,
-0.929781266907387));
#57661=CARTESIAN_POINT('Ctrl Pts',(-0.406550907978516,-0.0617095280149024,
-0.926180293360476));
#57662=CARTESIAN_POINT('Ctrl Pts',(-0.364609160678107,-0.257882177620295,
-0.914706856994306));
#57663=CARTESIAN_POINT('Ctrl Pts',(-0.0617202026280809,-0.475787586555369,
-0.895360957808874));
#57664=CARTESIAN_POINT('Ctrl Pts',(0.363681217312252,-0.31292041018399,
-0.871743569351098));
#57665=CARTESIAN_POINT('Ctrl Pts',(0.461252584696539,0.132019938055431,
-0.848126180893318));
#57666=CARTESIAN_POINT('Ctrl Pts',(0.14304097544786,0.4579546814661,-0.824508792435541));
#57667=CARTESIAN_POINT('Ctrl Pts',(-0.288287440300272,0.374153517030152,
-0.80172715444023));
#57668=CARTESIAN_POINT('Ctrl Pts',(-0.406697106371536,0.119357192848475,
-0.786817979264179));
#57669=CARTESIAN_POINT('Ctrl Pts',(-0.407517210131742,-0.000231984110039793,
-0.779781266907388));
#57670=CARTESIAN_POINT('Ctrl Pts',(-0.407484518933728,-0.000250174970737722,
-0.900218733092611));
#57671=CARTESIAN_POINT('Ctrl Pts',(-0.407598097974698,-0.0158774087335492,
-0.899299409193598));
#57672=CARTESIAN_POINT('Ctrl Pts',(-0.399732457373963,-0.16521027632643,
-0.890507622475326));
#57673=CARTESIAN_POINT('Ctrl Pts',(-0.215565140139133,-0.428619682337017,
-0.873843372937795));
#57674=CARTESIAN_POINT('Ctrl Pts',(0.239760820588477,-0.415569381260058,
-0.850225984480015));
#57675=CARTESIAN_POINT('Ctrl Pts',(0.478961233248966,-0.0279159233190857,
-0.826608596022238));
#57676=CARTESIAN_POINT('Ctrl Pts',(0.286415713505782,0.384901546875125,
-0.802991207564458));
#57677=CARTESIAN_POINT('Ctrl Pts',(-0.164311075821679,0.450760504139189,
-0.779373819106682));
#57678=CARTESIAN_POINT('Ctrl Pts',(-0.389705041663024,0.197172692304488,
-0.761782994282732));
#57679=CARTESIAN_POINT('Ctrl Pts',(-0.407325372263877,0.0318216989288424,
-0.752064632278042));
#57680=CARTESIAN_POINT('Ctrl Pts',(-0.407044529006025,0.000355972576201576,
-0.750218733092611));
#57681=CARTESIAN_POINT('Origin',(0.,0.,-1.90478126690739));
#57682=CARTESIAN_POINT('',(-0.407215026014371,0.000338947040179602,-1.07978126690739));
#57683=CARTESIAN_POINT('',(-0.406418685883609,-6.78377527379426E-5,-1.05021873309261));
#57684=CARTESIAN_POINT('',(-0.40705,-2.29167262861955E-14,-1.90478126690739));
#57685=CARTESIAN_POINT('Ctrl Pts',(-0.407215026014371,0.000338947040179598,
-1.07978126690739));
#57686=CARTESIAN_POINT('Ctrl Pts',(-0.40625104068007,-0.108064226981459,
-1.07341507027603));
#57687=CARTESIAN_POINT('Ctrl Pts',(-0.306311001088235,-0.352090017898099,
-1.05917641082542));
#57688=CARTESIAN_POINT('Ctrl Pts',(0.103992118918514,-0.468368284610657,
-1.03706528855554));
#57689=CARTESIAN_POINT('Ctrl Pts',(0.448505409809192,-0.170370503266186,
-1.01344790009777));
#57690=CARTESIAN_POINT('Ctrl Pts',(0.388726300769665,0.281202905405924,
-0.989830511639989));
#57691=CARTESIAN_POINT('Ctrl Pts',(-0.0214590362974804,0.479293981479854,
-0.96621312318221));
#57692=CARTESIAN_POINT('Ctrl Pts',(-0.35270860156304,0.281010568000828,
-0.946196708271343));
#57693=CARTESIAN_POINT('Ctrl Pts',(-0.40628027302014,0.0730034436260336,
-0.934052756179736));
#57694=CARTESIAN_POINT('Ctrl Pts',(-0.406427115799581,-8.99486733453581E-5,
-0.929781266907387));
#57695=CARTESIAN_POINT('Ctrl Pts',(-0.406418685883609,-6.78377527379634E-5,
-1.05021873309261));
#57696=CARTESIAN_POINT('Ctrl Pts',(-0.406514099565618,-0.0631207687989047,
-1.04653418610915));
#57697=CARTESIAN_POINT('Ctrl Pts',(-0.36319902856371,-0.260769488780026,
-1.03497717630644));
#57698=CARTESIAN_POINT('Ctrl Pts',(-0.0567200932042535,-0.476409480116128,
-1.01554770368446));
#57699=CARTESIAN_POINT('Ctrl Pts',(0.366947398132722,-0.309083756844029,
-0.991930315226685));
#57700=CARTESIAN_POINT('Ctrl Pts',(0.459840631415877,0.136856696679471,
-0.968312926768907));
#57701=CARTESIAN_POINT('Ctrl Pts',(0.138223653062154,0.459431587358633,
-0.944695538311129));
#57702=CARTESIAN_POINT('Ctrl Pts',(-0.290621860797603,0.371429283499432,
-0.921997473752364));
#57703=CARTESIAN_POINT('Ctrl Pts',(-0.40662548453775,0.11794356219702,-0.907171872012857));
#57704=CARTESIAN_POINT('Ctrl Pts',(-0.407484518933728,-0.000250174970737722,
-0.900218733092611));
#57705=CARTESIAN_POINT('Origin',(0.,0.,-1.90478126690739));
#57706=CARTESIAN_POINT('',(-0.407335136724506,-0.000310347641450006,-1.22978126690739));
#57707=CARTESIAN_POINT('',(-0.407256252750017,0.00033078647732554,-1.20021873309261));
#57708=CARTESIAN_POINT('',(-0.40705,-2.29167262861955E-14,-1.90478126690739));
#57709=CARTESIAN_POINT('Ctrl Pts',(-0.407335136724506,-0.000310347641449972,
-1.22978126690739));
#57710=CARTESIAN_POINT('Ctrl Pts',(-0.407516487490046,-0.0217313980275844,
-1.22852231001085));
#57711=CARTESIAN_POINT('Ctrl Pts',(-0.3962986870886,-0.176911566770959,
-1.21939089029505));
#57712=CARTESIAN_POINT('Ctrl Pts',(-0.19708110914224,-0.437426850444666,
-1.20238700775999));
#57713=CARTESIAN_POINT('Ctrl Pts',(0.257273433552846,-0.404961213377078,
-1.17876961930221));
#57714=CARTESIAN_POINT('Ctrl Pts',(0.47971620707788,-0.00745486488903116,
-1.15515223084444));
#57715=CARTESIAN_POINT('Ctrl Pts',(0.269732486126293,0.396771466717889,
-1.13153484238666));
#57716=CARTESIAN_POINT('Ctrl Pts',(-0.183393878810481,0.443339480829272,
-1.10791745392888));
#57717=CARTESIAN_POINT('Ctrl Pts',(-0.393623984240889,0.185443113339493,
-1.09066626210246));
#57718=CARTESIAN_POINT('Ctrl Pts',(-0.407443108588437,0.0259875477896631,
-1.08128753309529));
#57719=CARTESIAN_POINT('Ctrl Pts',(-0.407215026014371,0.000338947040179598,
-1.07978126690739));
#57720=CARTESIAN_POINT('Ctrl Pts',(-0.407256252750017,0.00033078647732554,
-1.20021873309261));
#57721=CARTESIAN_POINT('Ctrl Pts',(-0.406291321061865,-0.10946667159376,
-1.19376896302471));
#57722=CARTESIAN_POINT('Ctrl Pts',(-0.304151795041626,-0.354864242487783,
-1.17944673013755));
#57723=CARTESIAN_POINT('Ctrl Pts',(0.108905154226429,-0.467250284345138,
-1.15725203443113));
#57724=CARTESIAN_POINT('Ctrl Pts',(0.450269851614892,-0.165650906977965,
-1.13363464597335));
#57725=CARTESIAN_POINT('Ctrl Pts',(0.385751642062305,0.285269753596648,
-1.11001725751558));
#57726=CARTESIAN_POINT('Ctrl Pts',(-0.0264913736532199,0.479042136709866,
-1.0863998690578));
#57727=CARTESIAN_POINT('Ctrl Pts',(-0.354265995702489,0.278133272522654,
-1.06646702758348));
#57728=CARTESIAN_POINT('Ctrl Pts',(-0.406310237145777,0.0715991458975248,
-1.05440664892841));
#57729=CARTESIAN_POINT('Ctrl Pts',(-0.406418685883609,-6.78377527379634E-5,
-1.05021873309261));
#57730=CARTESIAN_POINT('Origin',(0.,0.,-1.90478126690739));
#57731=CARTESIAN_POINT('',(-0.406408689871578,2.35123281448032E-5,-1.37978126690739));
#57732=CARTESIAN_POINT('',(-0.407295256592268,-0.000321495865622912,-1.35021873309261));
#57733=CARTESIAN_POINT('',(-0.40705,-2.29167262861955E-14,-1.90478126690739));
#57734=CARTESIAN_POINT('Ctrl Pts',(-0.406408689871578,2.35123281448202E-5,
-1.37978126690739));
#57735=CARTESIAN_POINT('Ctrl Pts',(-0.406372411151293,-0.0688453689981078,
-1.37575708692641));
#57736=CARTESIAN_POINT('Ctrl Pts',(-0.357256431910931,-0.272490465756646,
-1.36386044412616));
#57737=CARTESIAN_POINT('Ctrl Pts',(-0.0363410200831963,-0.478396170765624,
-1.34409133850666));
#57738=CARTESIAN_POINT('Ctrl Pts',(0.379800489517723,-0.293145714789055,
-1.32047395004888));
#57739=CARTESIAN_POINT('Ctrl Pts',(0.453582904114614,0.156351802812663,
-1.2968565615911));
#57740=CARTESIAN_POINT('Ctrl Pts',(0.118495324937651,0.464910853754055,
-1.27323917313333));
#57741=CARTESIAN_POINT('Ctrl Pts',(-0.299849997018574,0.360280589402105,
-1.25088074157209));
#57742=CARTESIAN_POINT('Ctrl Pts',(-0.40638247157347,0.112217923969001,
-1.23639477283011));
#57743=CARTESIAN_POINT('Ctrl Pts',(-0.407335136724506,-0.000310347641449972,
-1.22978126690739));
#57744=CARTESIAN_POINT('Ctrl Pts',(-0.407295256592268,-0.000321495865622943,
-1.35021873309261));
#57745=CARTESIAN_POINT('Ctrl Pts',(-0.407492918321581,-0.0231703370026054,
-1.34887620275953));
#57746=CARTESIAN_POINT('Ctrl Pts',(-0.395411489547801,-0.179793560026876,
-1.33966120960718));
#57747=CARTESIAN_POINT('Ctrl Pts',(-0.192476314157182,-0.439472483121615,
-1.32257375363558));
#57748=CARTESIAN_POINT('Ctrl Pts',(0.26151206617616,-0.402236929927433,
-1.2989563651778));
#57749=CARTESIAN_POINT('Ctrl Pts',(0.479768010181106,-0.00241651336352132,
-1.27533897672002));
#57750=CARTESIAN_POINT('Ctrl Pts',(0.265550697114187,0.399582270810862,
-1.25172158826225));
#57751=CARTESIAN_POINT('Ctrl Pts',(-0.188039671187417,0.44138898578519,
-1.22810419980447));
#57752=CARTESIAN_POINT('Ctrl Pts',(-0.394544467466406,0.182559052872597,
-1.21093658141459));
#57753=CARTESIAN_POINT('Ctrl Pts',(-0.407469097751286,0.0245499518228972,
-1.20164142584397));
#57754=CARTESIAN_POINT('Ctrl Pts',(-0.407256252750017,0.00033078647732554,
-1.20021873309261));
#57755=CARTESIAN_POINT('Origin',(0.,0.,-1.90478126690739));
#57756=CARTESIAN_POINT('',(-0.407376298364278,0.000257087447545755,-1.52978126690739));
#57757=CARTESIAN_POINT('',(-0.406409642899809,4.34815695103397E-5,-1.50021873309261));
#57758=CARTESIAN_POINT('',(-0.40705,-2.29167262861955E-14,-1.90478126690739));
#57759=CARTESIAN_POINT('Ctrl Pts',(-0.407376298364278,0.00025708744754576,
-1.52978126690739));
#57760=CARTESIAN_POINT('Ctrl Pts',(-0.406454140896361,-0.115208344033967,
-1.52299186384196));
#57761=CARTESIAN_POINT('Ctrl Pts',(-0.295182303803987,-0.366031497986206,
-1.50832999795728));
#57762=CARTESIAN_POINT('Ctrl Pts',(0.128775427374938,-0.462199578908625,
-1.48579566925333));
#57763=CARTESIAN_POINT('Ctrl Pts',(0.456910236919244,-0.146277500967067,
-1.46217828079555));
#57764=CARTESIAN_POINT('Ctrl Pts',(0.373237957669861,0.301462946406964,
-1.43856089233778));
#57765=CARTESIAN_POINT('Ctrl Pts',(-0.046911046254029,0.477478658159383,
-1.41494350387999));
#57766=CARTESIAN_POINT('Ctrl Pts',(-0.360375435904293,0.266422351665797,
-1.3953502954032));
#57767=CARTESIAN_POINT('Ctrl Pts',(-0.406443382846875,0.0658821308172752,
-1.38362954974566));
#57768=CARTESIAN_POINT('Ctrl Pts',(-0.406408689871578,2.35123281448202E-5,
-1.37978126690739));
#57769=CARTESIAN_POINT('Ctrl Pts',(-0.406409642899809,4.34815695103258E-5,
-1.50021873309261));
#57770=CARTESIAN_POINT('Ctrl Pts',(-0.406338718852544,-0.0702526545189025,
-1.49611097967508));
#57771=CARTESIAN_POINT('Ctrl Pts',(-0.355745821427167,-0.275366303807096,
-1.4841307634383));
#57772=CARTESIAN_POINT('Ctrl Pts',(-0.0313114294066901,-0.478754704371251,
-1.46427808438225));
#57773=CARTESIAN_POINT('Ctrl Pts',(0.382856292689895,-0.28913914624985,
-1.44066069592447));
#57774=CARTESIAN_POINT('Ctrl Pts',(0.451916785881922,0.161105773860312,
-1.41704330746669));
#57775=CARTESIAN_POINT('Ctrl Pts',(0.113605814801219,0.466130064220589,
-1.39342591900891));
#57776=CARTESIAN_POINT('Ctrl Pts',(-0.302057329836814,0.357518966974991,
-1.37115106088422));
#57777=CARTESIAN_POINT('Ctrl Pts',(-0.406333849824981,0.110812968909595,
-1.35674866557879));
#57778=CARTESIAN_POINT('Ctrl Pts',(-0.407295256592268,-0.000321495865622943,
-1.35021873309261));
#57779=CARTESIAN_POINT('Origin',(0.,0.,2.85));
#57780=CARTESIAN_POINT('',(-9.49101269339199E-17,-0.458257569495584,1.3));
#57781=CARTESIAN_POINT('',(-1.53080849893419E-16,-6.12323399573677E-17,
1.6));
#57782=CARTESIAN_POINT('Origin',(-2.14313189850787E-16,0.,1.1));
#57783=CARTESIAN_POINT('',(0.367006645104718,-0.474664220738176,1.3));
#57784=CARTESIAN_POINT('Ctrl Pts',(0.367006645104718,-0.474664220738176,
1.3));
#57785=CARTESIAN_POINT('Ctrl Pts',(0.338138729685014,-0.47246220371005,
1.3));
#57786=CARTESIAN_POINT('Ctrl Pts',(0.309024935784566,-0.470333761200034,
1.3));
#57787=CARTESIAN_POINT('Ctrl Pts',(0.183814615587507,-0.462023903676248,
1.3));
#57788=CARTESIAN_POINT('Ctrl Pts',(0.0876016538044517,-0.458257569495584,
1.3));
#57789=CARTESIAN_POINT('Ctrl Pts',(0.,-0.458257569495584,1.3));
#57790=CARTESIAN_POINT('',(0.827500847770699,-0.194273896699414,0.8));
#57791=CARTESIAN_POINT('Ctrl Pts',(0.827500847770699,-0.194273896699415,
0.8));
#57792=CARTESIAN_POINT('Ctrl Pts',(0.806825653221766,-0.247573683077793,
0.815891726644921));
#57793=CARTESIAN_POINT('Ctrl Pts',(0.77844058049192,-0.295313715449721,
0.837983964638171));
#57794=CARTESIAN_POINT('Ctrl Pts',(0.70695573897281,-0.382945194539716,
0.896201780082199));
#57795=CARTESIAN_POINT('Ctrl Pts',(0.66279406000339,-0.420213839249111,
0.933475334456469));
#57796=CARTESIAN_POINT('Ctrl Pts',(0.568627272529482,-0.476124483335569,
1.02033912838166));
#57797=CARTESIAN_POINT('Ctrl Pts',(0.520183006714955,-0.492461401650283,
1.06898944325634));
#57798=CARTESIAN_POINT('Ctrl Pts',(0.448389981387326,-0.501794096344547,
1.15498482706113));
#57799=CARTESIAN_POINT('Ctrl Pts',(0.420349703511602,-0.500357460127172,
1.19326140983976));
#57800=CARTESIAN_POINT('Ctrl Pts',(0.385715038223485,-0.488539976457829,
1.25517036827747));
#57801=CARTESIAN_POINT('Ctrl Pts',(0.375253631229262,-0.482576530120786,
1.27739203707623));
#57802=CARTESIAN_POINT('Ctrl Pts',(0.367006645104718,-0.474664220738176,
1.3));
#57803=CARTESIAN_POINT('',(0.827500847770699,0.194273896699414,0.8));
#57804=CARTESIAN_POINT('Ctrl Pts',(0.827500847770699,0.194273896699414,
0.8));
#57805=CARTESIAN_POINT('Ctrl Pts',(0.832240686457716,0.190066469416246,
0.8));
#57806=CARTESIAN_POINT('Ctrl Pts',(0.83681804160594,0.185810667739891,0.8));
#57807=CARTESIAN_POINT('Ctrl Pts',(0.86737452556169,0.15603927066178,0.8));
#57808=CARTESIAN_POINT('Ctrl Pts',(0.893751654888157,0.121036696804236,
0.8));
#57809=CARTESIAN_POINT('Ctrl Pts',(0.919853574042595,0.0616080446153948,
0.8));
#57810=CARTESIAN_POINT('Ctrl Pts',(0.92736184954957,0.0283844942503903,
0.8));
#57811=CARTESIAN_POINT('Ctrl Pts',(0.92736184954957,-0.0283844942503903,
0.8));
#57812=CARTESIAN_POINT('Ctrl Pts',(0.919853574042595,-0.0616080446153948,
0.8));
#57813=CARTESIAN_POINT('Ctrl Pts',(0.893751654888157,-0.121036696804236,
0.8));
#57814=CARTESIAN_POINT('Ctrl Pts',(0.86737452556169,-0.15603927066178,0.8));
#57815=CARTESIAN_POINT('Ctrl Pts',(0.83681804160594,-0.185810667739891,
0.8));
#57816=CARTESIAN_POINT('Ctrl Pts',(0.832240686457716,-0.190066469416246,
0.8));
#57817=CARTESIAN_POINT('Ctrl Pts',(0.827500847770699,-0.194273896699414,
0.8));
#57818=CARTESIAN_POINT('',(0.367006645104718,0.474664220738176,1.3));
#57819=CARTESIAN_POINT('Ctrl Pts',(0.367006645104718,0.474664220738176,
1.3));
#57820=CARTESIAN_POINT('Ctrl Pts',(0.386844565037868,0.49369708409554,1.24561710768513));
#57821=CARTESIAN_POINT('Ctrl Pts',(0.416544185701006,0.498879203778029,
1.20057273466721));
#57822=CARTESIAN_POINT('Ctrl Pts',(0.471907063756615,0.501218135446952,
1.12399758848168));
#57823=CARTESIAN_POINT('Ctrl Pts',(0.51158524080212,0.49437132413065,1.07934345321278));
#57824=CARTESIAN_POINT('Ctrl Pts',(0.6046391383893,0.458711546216609,0.985187921540669));
#57825=CARTESIAN_POINT('Ctrl Pts',(0.657180998804381,0.425900587285382,
0.938631347135963));
#57826=CARTESIAN_POINT('Ctrl Pts',(0.728744413965246,0.357037429469063,
0.878319677166941));
#57827=CARTESIAN_POINT('Ctrl Pts',(0.751978600292447,0.32968521463109,0.859423759568972));
#57828=CARTESIAN_POINT('Ctrl Pts',(0.794210469526027,0.267260154796302,
0.825735732037567));
#57829=CARTESIAN_POINT('Ctrl Pts',(0.812815008506796,0.232133375781979,
0.811288084500528));
#57830=CARTESIAN_POINT('Ctrl Pts',(0.827500847770699,0.194273896699415,
0.8));
#57831=CARTESIAN_POINT('',(-6.7154551318291E-17,0.458257569495584,1.3));
#57832=CARTESIAN_POINT('Ctrl Pts',(5.55111512312578E-17,0.458257569495584,
1.3));
#57833=CARTESIAN_POINT('Ctrl Pts',(0.0876016538044517,0.458257569495584,
1.3));
#57834=CARTESIAN_POINT('Ctrl Pts',(0.183814615587507,0.462023903676248,
1.3));
#57835=CARTESIAN_POINT('Ctrl Pts',(0.309024935784565,0.470333761200034,
1.3));
#57836=CARTESIAN_POINT('Ctrl Pts',(0.338138729685014,0.47246220371005,1.3));
#57837=CARTESIAN_POINT('Ctrl Pts',(0.367006645104718,0.474664220738176,
1.3));
#57838=CARTESIAN_POINT('Origin',(-2.14313189850787E-16,0.,1.1));
#57839=CARTESIAN_POINT('Origin',(0.,-6.12323399573677E-17,2.85));
#57840=CARTESIAN_POINT('',(-0.367006645104718,0.474664220738176,1.3));
#57841=CARTESIAN_POINT('Ctrl Pts',(-0.367006645104718,0.474664220738176,
1.3));
#57842=CARTESIAN_POINT('Ctrl Pts',(-0.338138729685014,0.47246220371005,
1.3));
#57843=CARTESIAN_POINT('Ctrl Pts',(-0.309024935784565,0.470333761200034,
1.3));
#57844=CARTESIAN_POINT('Ctrl Pts',(-0.183814615587506,0.462023903676248,
1.3));
#57845=CARTESIAN_POINT('Ctrl Pts',(-0.0876016538044515,0.458257569495584,
1.3));
#57846=CARTESIAN_POINT('Ctrl Pts',(5.55111512312578E-17,0.458257569495584,
1.3));
#57847=CARTESIAN_POINT('',(-0.827500847770699,0.194273896699414,0.8));
#57848=CARTESIAN_POINT('Ctrl Pts',(-0.827500847770699,0.194273896699414,
0.8));
#57849=CARTESIAN_POINT('Ctrl Pts',(-0.806825653221767,0.247573683077793,
0.815891726644921));
#57850=CARTESIAN_POINT('Ctrl Pts',(-0.77844058049192,0.295313715449721,
0.837983964638171));
#57851=CARTESIAN_POINT('Ctrl Pts',(-0.706955738972811,0.382945194539717,
0.896201780082199));
#57852=CARTESIAN_POINT('Ctrl Pts',(-0.66279406000339,0.420213839249111,
0.933475334456469));
#57853=CARTESIAN_POINT('Ctrl Pts',(-0.56862727252948,0.476124483335571,
1.02033912838166));
#57854=CARTESIAN_POINT('Ctrl Pts',(-0.520183006714953,0.492461401650283,
1.06898944325634));
#57855=CARTESIAN_POINT('Ctrl Pts',(-0.448389981387328,0.501794096344547,
1.15498482706113));
#57856=CARTESIAN_POINT('Ctrl Pts',(-0.420349703511603,0.500357460127172,
1.19326140983976));
#57857=CARTESIAN_POINT('Ctrl Pts',(-0.385715038223483,0.488539976457828,
1.25517036827748));
#57858=CARTESIAN_POINT('Ctrl Pts',(-0.375253631229262,0.482576530120786,
1.27739203707623));
#57859=CARTESIAN_POINT('Ctrl Pts',(-0.367006645104718,0.474664220738176,
1.3));
#57860=CARTESIAN_POINT('',(-0.827500847770699,-0.194273896699414,0.8));
#57861=CARTESIAN_POINT('Ctrl Pts',(-0.827500847770699,-0.194273896699414,
0.8));
#57862=CARTESIAN_POINT('Ctrl Pts',(-0.832240686457716,-0.190066469416245,
0.8));
#57863=CARTESIAN_POINT('Ctrl Pts',(-0.83681804160594,-0.185810667739891,
0.8));
#57864=CARTESIAN_POINT('Ctrl Pts',(-0.86737452556169,-0.15603927066178,
0.8));
#57865=CARTESIAN_POINT('Ctrl Pts',(-0.893751654888157,-0.121036696804236,
0.8));
#57866=CARTESIAN_POINT('Ctrl Pts',(-0.919853574042595,-0.0616080446153948,
0.8));
#57867=CARTESIAN_POINT('Ctrl Pts',(-0.92736184954957,-0.0283844942503903,
0.8));
#57868=CARTESIAN_POINT('Ctrl Pts',(-0.92736184954957,0.0283844942503903,
0.8));
#57869=CARTESIAN_POINT('Ctrl Pts',(-0.919853574042595,0.0616080446153948,
0.8));
#57870=CARTESIAN_POINT('Ctrl Pts',(-0.893751654888157,0.121036696804236,
0.8));
#57871=CARTESIAN_POINT('Ctrl Pts',(-0.86737452556169,0.15603927066178,0.8));
#57872=CARTESIAN_POINT('Ctrl Pts',(-0.83681804160594,0.185810667739891,
0.8));
#57873=CARTESIAN_POINT('Ctrl Pts',(-0.832240686457716,0.190066469416246,
0.8));
#57874=CARTESIAN_POINT('Ctrl Pts',(-0.827500847770699,0.194273896699414,
0.8));
#57875=CARTESIAN_POINT('',(-0.367006645104718,-0.474664220738176,1.3));
#57876=CARTESIAN_POINT('Ctrl Pts',(-0.367006645104718,-0.474664220738176,
1.3));
#57877=CARTESIAN_POINT('Ctrl Pts',(-0.386844565037811,-0.493697084095486,
1.24561710768529));
#57878=CARTESIAN_POINT('Ctrl Pts',(-0.416544185700876,-0.498879203778024,
1.20057273466739));
#57879=CARTESIAN_POINT('Ctrl Pts',(-0.471907063756621,-0.501218135446952,
1.12399758848167));
#57880=CARTESIAN_POINT('Ctrl Pts',(-0.511585240802128,-0.494371324130647,
1.07934345321277));
#57881=CARTESIAN_POINT('Ctrl Pts',(-0.6046391383893,-0.458711546216609,
0.98518792154067));
#57882=CARTESIAN_POINT('Ctrl Pts',(-0.657180998804382,-0.425900587285382,
0.938631347135963));
#57883=CARTESIAN_POINT('Ctrl Pts',(-0.728744413965246,-0.357037429469062,
0.878319677166941));
#57884=CARTESIAN_POINT('Ctrl Pts',(-0.751978600292447,-0.32968521463109,
0.859423759568971));
#57885=CARTESIAN_POINT('Ctrl Pts',(-0.794210469526026,-0.267260154796303,
0.825735732037568));
#57886=CARTESIAN_POINT('Ctrl Pts',(-0.812815008506795,-0.232133375781979,
0.811288084500528));
#57887=CARTESIAN_POINT('Ctrl Pts',(-0.827500847770699,-0.194273896699414,
0.8));
#57888=CARTESIAN_POINT('Ctrl Pts',(0.,-0.458257569495584,1.3));
#57889=CARTESIAN_POINT('Ctrl Pts',(-0.0876016538044516,-0.458257569495584,
1.3));
#57890=CARTESIAN_POINT('Ctrl Pts',(-0.183814615587506,-0.462023903676248,
1.3));
#57891=CARTESIAN_POINT('Ctrl Pts',(-0.309024935784565,-0.470333761200034,
1.3));
#57892=CARTESIAN_POINT('Ctrl Pts',(-0.338138729685014,-0.47246220371005,
1.3));
#57893=CARTESIAN_POINT('Ctrl Pts',(-0.367006645104718,-0.474664220738176,
1.3));
#57894=CARTESIAN_POINT('Origin',(0.,0.,0.8));
#57895=CARTESIAN_POINT('',(-1.05,-1.28587913910472E-16,0.8));
#57896=CARTESIAN_POINT('Origin',(0.,0.,0.8));
#57897=CARTESIAN_POINT('Origin',(0.,0.,0.8));
#57898=CARTESIAN_POINT('Origin',(0.,0.,0.8));
#57899=CARTESIAN_POINT('Origin',(0.,0.,1.3));
#57900=CARTESIAN_POINT('Origin',(0.,0.,1.3));
#57901=CARTESIAN_POINT('Origin',(0.,0.,1.));
#57902=CARTESIAN_POINT('Origin',(0.,0.,1.));
#57903=CARTESIAN_POINT('Origin',(0.,0.,1.3));
#57904=CARTESIAN_POINT('Origin',(0.,0.,1.3));
#57905=CARTESIAN_POINT('Origin',(1.25,0.,0.));
#57906=CARTESIAN_POINT('',(-1.25,-1.53080849893419E-16,0.));
#57907=CARTESIAN_POINT('Origin',(0.,0.,0.));
#57908=CARTESIAN_POINT('',(0.230288547470477,0.435342893480459,0.));
#57909=CARTESIAN_POINT('Ctrl Pts',(-0.407032914766026,-0.00372944996921218,
2.22044604925031E-16));
#57910=CARTESIAN_POINT('Ctrl Pts',(-0.409502406107154,0.0185484342735974,
1.33393110592597E-16));
#57911=CARTESIAN_POINT('Ctrl Pts',(-0.410064146186531,0.0409298249901961,
6.41710304853556E-17));
#57912=CARTESIAN_POINT('Ctrl Pts',(-0.408816203516182,0.0632211419519473,
-2.58907478789538E-16));
#57913=CARTESIAN_POINT('Ctrl Pts',(-0.408113237416965,0.0757778406716244,
-4.40897601254181E-16));
#57914=CARTESIAN_POINT('Ctrl Pts',(-0.406835127950302,0.0883063527932494,
-1.57466213752448E-16));
#57915=CARTESIAN_POINT('Ctrl Pts',(-0.404992377388169,0.100773692152307,
-6.07153216591882E-18));
#57916=CARTESIAN_POINT('Ctrl Pts',(-0.404012526054069,0.107402988246245,
7.44300201204056E-17));
#57917=CARTESIAN_POINT('Ctrl Pts',(-0.402873550921039,0.114009987474989,
-1.14344253592689E-16));
#57918=CARTESIAN_POINT('Ctrl Pts',(-0.401579163263675,0.120581758409531,
-1.8474805019153E-16));
#57919=CARTESIAN_POINT('Ctrl Pts',(-0.397116077809508,0.143241411488897,
-4.2750234310436E-16));
#57920=CARTESIAN_POINT('Ctrl Pts',(-0.390805198236086,0.165510695939246,
-2.33788451815087E-16));
#57921=CARTESIAN_POINT('Ctrl Pts',(-0.38271795691015,0.187189446898724,
-2.74086309204336E-16));
#57922=CARTESIAN_POINT('Ctrl Pts',(-0.381208311546034,0.191236219409497,
-2.81608710371759E-16));
#57923=CARTESIAN_POINT('Ctrl Pts',(-0.379636621493342,0.195262415265924,
-3.76247800759317E-16));
#57924=CARTESIAN_POINT('Ctrl Pts',(-0.378003151308578,0.199266719882105,
-4.02455846426619E-16));
#57925=CARTESIAN_POINT('Ctrl Pts',(-0.374957182270889,0.206733637853503,
-4.54796032731822E-16));
#57926=CARTESIAN_POINT('Ctrl Pts',(-0.371694472063554,0.214127904294756,
-6.04095780210171E-16));
#57927=CARTESIAN_POINT('Ctrl Pts',(-0.368232811861738,0.221415799627647,
-6.38378239159465E-16));
#57928=CARTESIAN_POINT('Ctrl Pts',(-0.358129974694566,0.242685483983424,
-7.38431416034905E-16));
#57929=CARTESIAN_POINT('Ctrl Pts',(-0.346322064408441,0.263089787169291,
-3.51612244000906E-16));
#57930=CARTESIAN_POINT('Ctrl Pts',(-0.332976726379132,0.282417007099477,
-3.19189119579733E-16));
#57931=CARTESIAN_POINT('Ctrl Pts',(-0.321328421888677,0.299286519299645,
-2.90889017704434E-16));
#57932=CARTESIAN_POINT('Ctrl Pts',(-0.308507716760313,0.315336147391315,
-2.43035058606971E-16));
#57933=CARTESIAN_POINT('Ctrl Pts',(-0.294595609651327,0.330416226174529,
-5.55111512312578E-17));
#57934=CARTESIAN_POINT('Ctrl Pts',(-0.289438034934074,0.33600679793028,
1.40087680724686E-17));
#57935=CARTESIAN_POINT('Ctrl Pts',(-0.28413020536853,0.341463974937307,
-3.4552926784595E-16));
#57936=CARTESIAN_POINT('Ctrl Pts',(-0.278675394220103,0.346779509590223,
-3.78169717762944E-16));
#57937=CARTESIAN_POINT('Ctrl Pts',(-0.2742428149802,0.351098912757517,-4.04693345574494E-16));
#57938=CARTESIAN_POINT('Ctrl Pts',(-0.269718867723713,0.355319082487331,
-7.06198858179791E-16));
#57939=CARTESIAN_POINT('Ctrl Pts',(-0.265111332520466,0.359431662343205,
-7.11236625150491E-16));
#57940=CARTESIAN_POINT('Ctrl Pts',(-0.260094342853417,0.363909711827728,
-7.16722079677064E-16));
#57941=CARTESIAN_POINT('Ctrl Pts',(-0.254976429475008,0.368261987646387,
-1.0019210278739E-16));
#57942=CARTESIAN_POINT('Ctrl Pts',(-0.249761050372628,0.372483785414168,
-1.2490009027033E-16));
#57943=CARTESIAN_POINT('Ctrl Pts',(-0.231304668403533,0.387424043958917,
-2.15807103259361E-16));
#57944=CARTESIAN_POINT('Ctrl Pts',(-0.211631027480377,0.40073306681961,
-3.74687250457173E-16));
#57945=CARTESIAN_POINT('Ctrl Pts',(-0.190986132226159,0.412423252290443,
-5.72458747072346E-16));
#57946=CARTESIAN_POINT('Ctrl Pts',(-0.176606675051318,0.420565629341712,
-7.10209349870931E-16));
#57947=CARTESIAN_POINT('Ctrl Pts',(-0.161754960911602,0.427921985785738,
-3.10111003734457E-16));
#57948=CARTESIAN_POINT('Ctrl Pts',(-0.146504136099264,0.434485677558816,
-2.32452945780892E-16));
#57949=CARTESIAN_POINT('Ctrl Pts',(-0.141356939441595,0.436700942160703,
-2.06243130819525E-16));
#57950=CARTESIAN_POINT('Ctrl Pts',(-0.136164227967783,0.438825835570468,
-2.69285390156797E-16));
#57951=CARTESIAN_POINT('Ctrl Pts',(-0.130928672659677,0.440859850121791,
-2.81025203108243E-16));
#57952=CARTESIAN_POINT('Ctrl Pts',(-0.12556463322452,0.442943780788724,
-2.93053119141415E-16));
#57953=CARTESIAN_POINT('Ctrl Pts',(-0.120163646959754,0.444929160518309,
1.39490241327531E-16));
#57954=CARTESIAN_POINT('Ctrl Pts',(-0.114731899809621,0.446815240591704,
8.32667268468867E-17));
#57955=CARTESIAN_POINT('Ctrl Pts',(-0.090250938166801,0.455315830301767,
-1.70133452392181E-16));
#57956=CARTESIAN_POINT('Ctrl Pts',(-0.0651300509740424,0.461810294150359,
-3.06185542203807E-16));
#57957=CARTESIAN_POINT('Ctrl Pts',(-0.0396563962731094,0.466299278577248,
-1.45716771982052E-16));
#57958=CARTESIAN_POINT('Ctrl Pts',(-0.0205511552474096,0.469666016897415,
-2.53651943157355E-17));
#57959=CARTESIAN_POINT('Ctrl Pts',(-0.00124630488774171,0.471903779543234,
2.41706311978087E-16));
#57960=CARTESIAN_POINT('Ctrl Pts',(0.0181468923706612,0.472993406137991,
3.2612801348364E-16));
#57961=CARTESIAN_POINT('Ctrl Pts',(0.0255821880205217,0.473411165817946,
3.58495049284613E-16));
#57962=CARTESIAN_POINT('Ctrl Pts',(0.0330305209702806,0.473659971890404,
-9.54367323080526E-17));
#57963=CARTESIAN_POINT('Ctrl Pts',(0.040485736875469,0.473738030558778,
-8.32667268468867E-17));
#57964=CARTESIAN_POINT('Ctrl Pts',(0.0468700728995737,0.473804876747384,
-7.28448416503496E-17));
#57965=CARTESIAN_POINT('Ctrl Pts',(0.0532608144088334,0.473746273409567,
-2.22757456392369E-16));
#57966=CARTESIAN_POINT('Ctrl Pts',(0.0596358754189341,0.473561936641337,
-2.08166817117217E-16));
#57967=CARTESIAN_POINT('Ctrl Pts',(0.0853914116867899,0.47281720771841,
-1.49219971208295E-16));
#57968=CARTESIAN_POINT('Ctrl Pts',(0.110956177502877,0.470026036127248,
2.37366919974466E-16));
#57969=CARTESIAN_POINT('Ctrl Pts',(0.136073147414297,0.465167209120457,
-2.08166817117217E-17));
#57970=CARTESIAN_POINT('Ctrl Pts',(0.15428584587622,0.461643999455222,-2.08029554200206E-16));
#57971=CARTESIAN_POINT('Ctrl Pts',(0.172263718537645,0.457032689199025,
-3.38570523553356E-16));
#57972=CARTESIAN_POINT('Ctrl Pts',(0.18991046284926,0.451308070908747,-3.05311331771918E-16));
#57973=CARTESIAN_POINT('Ctrl Pts',(0.203544498658142,0.446885178539278,
-2.79614976471743E-16));
#57974=CARTESIAN_POINT('Ctrl Pts',(0.216980922989279,0.44179740741506,-4.64126606240054E-17));
#57975=CARTESIAN_POINT('Ctrl Pts',(0.230193623813293,0.436078300125993,
-2.08166817117217E-17));
#57976=CARTESIAN_POINT('',(0.485198770445679,0.0844890712341007,0.));
#57977=CARTESIAN_POINT('Ctrl Pts',(0.485198770445679,0.0844890712341024,
0.));
#57978=CARTESIAN_POINT('Ctrl Pts',(0.487483556903401,0.0587811609303886,
-3.6403309418082E-17));
#57979=CARTESIAN_POINT('Ctrl Pts',(0.487669957905918,0.032999272007226,
-2.16332978629155E-16));
#57980=CARTESIAN_POINT('Ctrl Pts',(0.48581703237745,0.0073557324105081,
2.10335221462188E-16));
#57981=CARTESIAN_POINT('Ctrl Pts',(0.484978594933728,-0.00424781206935033,
4.03399966647938E-16));
#57982=CARTESIAN_POINT('Ctrl Pts',(0.483721893431401,-0.0158229198346243,
2.67290005872947E-16));
#57983=CARTESIAN_POINT('Ctrl Pts',(0.482049056063943,-0.0273488775086491,
3.18321757841744E-16));
#57984=CARTESIAN_POINT('Ctrl Pts',(0.480594436537202,-0.0373713001440821,
3.62696533502297E-16));
#57985=CARTESIAN_POINT('Ctrl Pts',(0.478823707565005,-0.0473618152739592,
2.79537773708781E-16));
#57986=CARTESIAN_POINT('Ctrl Pts',(0.476744474029188,-0.0572755363954163,
2.58473797920544E-16));
#57987=CARTESIAN_POINT('Ctrl Pts',(0.471567675914175,-0.0819583495235461,
2.06029496558142E-16));
#57988=CARTESIAN_POINT('Ctrl Pts',(0.464479206920196,-0.106198761077193,
1.05439529942102E-16));
#57989=CARTESIAN_POINT('Ctrl Pts',(0.455507744329332,-0.129784129861741,
-2.60208521396521E-17));
#57990=CARTESIAN_POINT('Ctrl Pts',(0.453016977318907,-0.136332187985184,
-6.25184889018675E-17));
#57991=CARTESIAN_POINT('Ctrl Pts',(0.450380803012963,-0.142829602956097,
3.48322078259034E-16));
#57992=CARTESIAN_POINT('Ctrl Pts',(0.447599240832732,-0.149271416802534,
3.17454396103756E-16));
#57993=CARTESIAN_POINT('Ctrl Pts',(0.444098051027165,-0.157379814712454,
2.80213370992714E-16));
#57994=CARTESIAN_POINT('Ctrl Pts',(0.440363895277044,-0.16540477046754,
8.12677602785049E-16));
#57995=CARTESIAN_POINT('Ctrl Pts',(0.436415237431444,-0.173307069589165,
7.52869988573934E-16));
#57996=CARTESIAN_POINT('Ctrl Pts',(0.425357271841625,-0.195436956549305,
5.8538256225953E-16));
#57997=CARTESIAN_POINT('Ctrl Pts',(0.412606104374067,-0.216645497952098,
-5.94784681012512E-16));
#57998=CARTESIAN_POINT('Ctrl Pts',(0.398278421228196,-0.236702761090162,
-3.67761376907083E-16));
#57999=CARTESIAN_POINT('Ctrl Pts',(0.385785090947335,-0.25419212139795,
-1.69803543057391E-16));
#58000=CARTESIAN_POINT('Ctrl Pts',(0.372092020529464,-0.270806277051948,
4.79495696309758E-17));
#58001=CARTESIAN_POINT('Ctrl Pts',(0.357255291902388,-0.286367384027322,
-3.46944695195361E-17));
#58002=CARTESIAN_POINT('Ctrl Pts',(0.351948789708481,-0.291932967275489,
-6.42529244922329E-17));
#58003=CARTESIAN_POINT('Ctrl Pts',(0.346495839949595,-0.297363574914842,
-1.69058141018443E-18));
#58004=CARTESIAN_POINT('Ctrl Pts',(0.340898563514322,-0.302650088761903,
4.16333634234434E-17));
#58005=CARTESIAN_POINT('Ctrl Pts',(0.336804911074738,-0.3065164603012,7.33189831192914E-17));
#58006=CARTESIAN_POINT('Ctrl Pts',(0.332634530931966,-0.31030506503389,
6.30416444442976E-17));
#58007=CARTESIAN_POINT('Ctrl Pts',(0.32839819773127,-0.314004190957375,
1.73472347597681E-17));
#58008=CARTESIAN_POINT('Ctrl Pts',(0.322231718417059,-0.319388702138902,
-4.91663322203621E-17));
#58009=CARTESIAN_POINT('Ctrl Pts',(0.315920306588548,-0.324588673796501,
-6.16839946309463E-17));
#58010=CARTESIAN_POINT('Ctrl Pts',(0.309467897502568,-0.329595262505712,
-4.16333634234434E-17));
#58011=CARTESIAN_POINT('Ctrl Pts',(0.2903984307146,-0.34439174794845,1.29797962091697E-17));
#58012=CARTESIAN_POINT('Ctrl Pts',(0.270098895473702,-0.357502851052604,
2.59113934393091E-17));
#58013=CARTESIAN_POINT('Ctrl Pts',(0.248817934772457,-0.368892164122873,
7.97972798949331E-17));
#58014=CARTESIAN_POINT('Ctrl Pts',(0.235636505678278,-0.375946705728147,
1.131742031205E-16));
#58015=CARTESIAN_POINT('Ctrl Pts',(0.222078033344231,-0.382339701258627,
2.48960342182608E-16));
#58016=CARTESIAN_POINT('Ctrl Pts',(0.208199770326819,-0.388052725523839,
1.73472347597681E-16));
#58017=CARTESIAN_POINT('Ctrl Pts',(0.202217607700804,-0.390515298844289,
1.40933588290973E-16));
#58018=CARTESIAN_POINT('Ctrl Pts',(0.196176028138775,-0.392851437390717,
7.6873750064169E-17));
#58019=CARTESIAN_POINT('Ctrl Pts',(0.190079662327023,-0.395059224742947,
6.93889390390723E-17));
#58020=CARTESIAN_POINT('Ctrl Pts',(0.184991168671714,-0.39690201309932,
6.31415427068228E-17));
#58021=CARTESIAN_POINT('Ctrl Pts',(0.179873425524456,-0.398652142795515,
3.22125190683935E-16));
#58022=CARTESIAN_POINT('Ctrl Pts',(0.174729796135838,-0.400309233186663,
3.2612801348364E-16));
#58023=CARTESIAN_POINT('Ctrl Pts',(0.152320431852445,-0.407528715661023,
3.43567200389085E-16));
#58024=CARTESIAN_POINT('Ctrl Pts',(0.129416852758522,-0.412987388760869,
3.861200852693E-16));
#58025=CARTESIAN_POINT('Ctrl Pts',(0.106249389798624,-0.41663803834582,
1.94289029309402E-16));
#58026=CARTESIAN_POINT('Ctrl Pts',(0.0893279915812928,-0.419304454408977,
5.41765925714067E-17));
#58027=CARTESIAN_POINT('Ctrl Pts',(0.0722654389196746,-0.421005297656241,
-2.92341994274838E-16));
#58028=CARTESIAN_POINT('Ctrl Pts',(0.0551537264920908,-0.421704837827871,
-4.02455846426619E-16));
#58029=CARTESIAN_POINT('Ctrl Pts',(0.0458345023082366,-0.422085814992642,
-4.62425044617213E-16));
#58030=CARTESIAN_POINT('Ctrl Pts',(0.0365007667942034,-0.422169548039371,
2.12962436588982E-16));
#58031=CARTESIAN_POINT('Ctrl Pts',(0.0271681775545658,-0.42194840310141,
2.0122792321331E-16));
#58032=CARTESIAN_POINT('Ctrl Pts',(0.021361805766906,-0.421810815375669,
1.93927168229147E-16));
#58033=CARTESIAN_POINT('Ctrl Pts',(0.0155642672926311,-0.421555318758217,
9.02804926475444E-17));
#58034=CARTESIAN_POINT('Ctrl Pts',(0.00978415844817893,-0.421181351844719,
5.55111512312578E-17));
#58035=CARTESIAN_POINT('Ctrl Pts',(-0.0123651918621571,-0.419748312364936,
-7.77248039753947E-17));
#58036=CARTESIAN_POINT('Ctrl Pts',(-0.0342836622346571,-0.416578763165458,
1.73036456657562E-16));
#58037=CARTESIAN_POINT('Ctrl Pts',(-0.0557672279919517,-0.411605196435151,
9.71445146547012E-17));
#58038=CARTESIAN_POINT('Ctrl Pts',(-0.069304109276844,-0.408471332012863,
4.93246964281187E-17));
#58039=CARTESIAN_POINT('Ctrl Pts',(-0.0826681142898227,-0.404620280484352,
7.89361148452016E-17));
#58040=CARTESIAN_POINT('Ctrl Pts',(-0.0958034133885173,-0.400025521834758,
1.38777878078145E-17));
#58041=CARTESIAN_POINT('Ctrl Pts',(-0.107098233124042,-0.396074567213513,
-4.9003652258222E-17));
#58042=CARTESIAN_POINT('Ctrl Pts',(-0.118223898010513,-0.39157345838643,
5.62305508459485E-18));
#58043=CARTESIAN_POINT('Ctrl Pts',(-0.129150719006634,-0.38654594480115,
-6.93889390390723E-18));
#58044=CARTESIAN_POINT('Origin',(0.,0.,0.));
#58045=CARTESIAN_POINT('Origin',(0.,0.,0.3));
#58046=CARTESIAN_POINT('',(-1.25,-1.53080849893419E-16,0.6));
#58047=CARTESIAN_POINT('Origin',(0.,0.,0.6));
#58048=CARTESIAN_POINT('',(-1.25,-1.53080849893419E-16,0.3));
#58049=CARTESIAN_POINT('Origin',(0.,0.,0.7));
#58050=CARTESIAN_POINT('',(-1.15,-1.40834381901946E-16,0.7));
#58051=CARTESIAN_POINT('Ctrl Pts',(0.285821514250011,-0.40107644158169,
-1.67683458050225));
#58052=CARTESIAN_POINT('Ctrl Pts',(0.351951188739807,-0.35395005433991,
-1.67289834909262));
#58053=CARTESIAN_POINT('Ctrl Pts',(0.459413146959217,-0.226542587597284,
-1.66502588627336));
#58054=CARTESIAN_POINT('Ctrl Pts',(0.532521434237499,0.101635635160784,
-1.64928096063485));
#58055=CARTESIAN_POINT('Ctrl Pts',(0.300949767170296,0.496361842456049,
-1.6295998035867));
#58056=CARTESIAN_POINT('Ctrl Pts',(-0.250382990617479,0.524039845133421,
-1.60598241512892));
#58057=CARTESIAN_POINT('Ctrl Pts',(-0.574972636888615,0.078666076090792,
-1.58236502667114));
#58058=CARTESIAN_POINT('Ctrl Pts',(-0.381802551317379,-0.437278299044204,
-1.55874763821336));
#58059=CARTESIAN_POINT('Ctrl Pts',(0.155808618062042,-0.559226858156241,
-1.53513024975558));
#58060=CARTESIAN_POINT('Ctrl Pts',(0.552827150676151,-0.176984815689186,
-1.51151286129781));
#58061=CARTESIAN_POINT('Ctrl Pts',(0.45158996229556,0.364747576723814,-1.48789547284003));
#58062=CARTESIAN_POINT('Ctrl Pts',(-0.0567588509522337,0.577713399197876,
-1.46427808438225));
#58063=CARTESIAN_POINT('Ctrl Pts',(-0.513923878567292,0.269903117161945,
-1.44066069592447));
#58064=CARTESIAN_POINT('Ctrl Pts',(-0.507837364089479,-0.281196945664769,
-1.41704330746669));
#58065=CARTESIAN_POINT('Ctrl Pts',(-0.0439699112909389,-0.578823520702787,
-1.39342591900891));
#58066=CARTESIAN_POINT('Ctrl Pts',(0.459530134105091,-0.354684349671076,
-1.36980853055114));
#58067=CARTESIAN_POINT('Ctrl Pts',(0.548801327297502,0.189173966061256,
-1.34619114209336));
#58068=CARTESIAN_POINT('Ctrl Pts',(0.143370464394534,0.562507297565094,
-1.32257375363558));
#58069=CARTESIAN_POINT('Ctrl Pts',(-0.391297213964002,0.428784228150806,
-1.2989563651778));
#58070=CARTESIAN_POINT('Ctrl Pts',(-0.57324139440495,-0.0914540128567207,
-1.27533897672002));
#58071=CARTESIAN_POINT('Ctrl Pts',(-0.238453374898797,-0.529253712919782,
-1.25172158826224));
#58072=CARTESIAN_POINT('Ctrl Pts',(0.311281577262681,-0.489972724697733,
-1.22810419980447));
#58073=CARTESIAN_POINT('Ctrl Pts',(0.58042066573113,-0.00901982792740492,
-1.20448681134669));
#58074=CARTESIAN_POINT('Ctrl Pts',(0.326356097327604,0.480063744892664,
-1.18086942288891));
#58075=CARTESIAN_POINT('Ctrl Pts',(-0.221892851772901,0.53640755265549,
-1.15725203443113));
#58076=CARTESIAN_POINT('Ctrl Pts',(-0.570122827353299,0.109222085715003,
-1.13363464597335));
#58077=CARTESIAN_POINT('Ctrl Pts',(-0.404431851492691,-0.416418514146393,
-1.11001725751558));
#58078=CARTESIAN_POINT('Ctrl Pts',(0.125822671827455,-0.566690529838469,
-1.0863998690578));
#58079=CARTESIAN_POINT('Ctrl Pts',(0.542657939641386,-0.206135543197639,
-1.06278248060002));
#58080=CARTESIAN_POINT('Ctrl Pts',(0.470329696914535,0.34023444518466,-1.03916509214224));
#58081=CARTESIAN_POINT('Ctrl Pts',(-0.025963826007878,0.579909804394615,
-1.01554770368446));
#58082=CARTESIAN_POINT('Ctrl Pts',(-0.498852999158645,0.296842023235613,
-0.991930315226685));
#58083=CARTESIAN_POINT('Ctrl Pts',(-0.52206537526902,-0.253805526836494,
-0.968312926768907));
#58084=CARTESIAN_POINT('Ctrl Pts',(-0.0746768205240931,-0.57566732926795,
-0.944695538311129));
#58085=CARTESIAN_POINT('Ctrl Pts',(0.440027022543379,-0.378610249393483,
-0.921078149853351));
#58086=CARTESIAN_POINT('Ctrl Pts',(0.558081066117299,0.1597342328763,-0.897460761395573));
#58087=CARTESIAN_POINT('Ctrl Pts',(0.173068862321762,0.554090850318274,
-0.873843372937794));
#58088=CARTESIAN_POINT('Ctrl Pts',(-0.367951327395403,0.448978086525479,
-0.850225984480016));
#58089=CARTESIAN_POINT('Ctrl Pts',(-0.577292295711129,-0.060853157885975,
-0.826608596022237));
#58090=CARTESIAN_POINT('Ctrl Pts',(-0.2662496020955,-0.515830060093211,
-0.802991207564461));
#58091=CARTESIAN_POINT('Ctrl Pts',(0.28479619558802,-0.505826678309667,
-0.77937381910668));
#58092=CARTESIAN_POINT('Ctrl Pts',(0.579120591889377,-0.039860275511877,
-0.755756430648904));
#58093=CARTESIAN_POINT('Ctrl Pts',(0.351413260849551,0.462037034889159,
-0.732139042191124));
#58094=CARTESIAN_POINT('Ctrl Pts',(-0.193065523547594,0.547444248416976,
-0.708521653733348));
#58095=CARTESIAN_POINT('Ctrl Pts',(-0.563510902565598,0.139373470280007,
-0.684904265275568));
#58096=CARTESIAN_POINT('Ctrl Pts',(-0.425995463083871,-0.394331544421604,
-0.661286876817791));
#58097=CARTESIAN_POINT('Ctrl Pts',(0.095521427029711,-0.572577644051913,
-0.637669488360011));
#58098=CARTESIAN_POINT('Ctrl Pts',(0.530933253458391,-0.234689969954635,
-0.614052099902234));
#58099=CARTESIAN_POINT('Ctrl Pts',(0.487750452992866,0.314752278720359,
-0.590434711444455));
#58100=CARTESIAN_POINT('Ctrl Pts',(0.00489892952646269,0.580470069784127,
-0.566817322986678));
#58101=CARTESIAN_POINT('Ctrl Pts',(-0.482368595405421,0.322939685458225,
-0.543199934528898));
#58102=CARTESIAN_POINT('Ctrl Pts',(-0.534818716119646,-0.225695460968752,
-0.519582546071121));
#58103=CARTESIAN_POINT('Ctrl Pts',(-0.105171775600954,-0.570883875267303,
-0.495965157613343));
#58104=CARTESIAN_POINT('Ctrl Pts',(0.419279269138383,-0.401465317274596,
-0.472347769155565));
#58105=CARTESIAN_POINT('Ctrl Pts',(0.565782966987249,0.129842695435552,
-0.448730380697786));
#58106=CARTESIAN_POINT('Ctrl Pts',(0.202277792416376,0.544107709314211,
-0.425112992240008));
#58107=CARTESIAN_POINT('Ctrl Pts',(-0.343564989114983,0.467902373344431,
-0.40149560378223));
#58108=CARTESIAN_POINT('Ctrl Pts',(-0.579710793277147,-0.0300802281383343,
-0.377878215324452));
#58109=CARTESIAN_POINT('Ctrl Pts',(-0.293293089483625,-0.500947815182221,
-0.354260826866673));
#58110=CARTESIAN_POINT('Ctrl Pts',(0.257505759040535,-0.520250391965063,
-0.330643438408895));
#58111=CARTESIAN_POINT('Ctrl Pts',(0.576182504633862,-0.0705879126061006,
-0.307026049951117));
#58112=CARTESIAN_POINT('Ctrl Pts',(0.375477683372268,0.442703659920605,
-0.283408661493339));
#58113=CARTESIAN_POINT('Ctrl Pts',(-0.163694059152507,0.556933358324603,
-0.259791273035561));
#58114=CARTESIAN_POINT('Ctrl Pts',(-0.555302152523182,0.169130024000774,
-0.236173884577782));
#58115=CARTESIAN_POINT('Ctrl Pts',(-0.446361113399504,-0.371128138543734,
-0.212556496120004));
#58116=CARTESIAN_POINT('Ctrl Pts',(0.0649627696741521,-0.576848443985302,
-0.188939107662226));
#58117=CARTESIAN_POINT('Ctrl Pts',(0.517682881343619,-0.262575546982227,
-0.165321719204448));
#58118=CARTESIAN_POINT('Ctrl Pts',(0.503838986030669,0.288370040921889,
-0.141704330746669));
#58119=CARTESIAN_POINT('Ctrl Pts',(0.0356574830697532,0.579408355918849,
-0.118086942288891));
#58120=CARTESIAN_POINT('Ctrl Pts',(-0.464346188869441,0.348086916704139,
-0.0944695538311128));
#58121=CARTESIAN_POINT('Ctrl Pts',(-0.54639681349325,-0.196875400907364,
-0.0708521653733346));
#58122=CARTESIAN_POINT('Ctrl Pts',(-0.134700387395815,-0.564625226713823,
-0.0472347769155564));
#58123=CARTESIAN_POINT('Ctrl Pts',(0.307439751116493,-0.44653071528208,
-0.0275536198674081));
#58124=CARTESIAN_POINT('Ctrl Pts',(0.486049448357886,-0.161672252861274,
-0.0118086942288891));
#58125=CARTESIAN_POINT('Ctrl Pts',(0.499129368704262,0.0044892671421744,
-0.00393623140962979));
#58126=CARTESIAN_POINT('Ctrl Pts',(0.485198770445679,0.0844890712341024,
0.));
#58127=CARTESIAN_POINT('Ctrl Pts',(0.269291261530782,-0.377880514723377,
-1.66038972033484));
#58128=CARTESIAN_POINT('Ctrl Pts',(0.331596380565313,-0.333479643413787,
-1.65645348892521));
#58129=CARTESIAN_POINT('Ctrl Pts',(0.432843364619005,-0.213440682954178,
-1.64858102610595));
#58130=CARTESIAN_POINT('Ctrl Pts',(0.501723494098348,0.0957576216078316,
-1.63283610046743));
#58131=CARTESIAN_POINT('Ctrl Pts',(0.283544584358314,0.467655162633464,
-1.61315494341928));
#58132=CARTESIAN_POINT('Ctrl Pts',(-0.235902295830161,0.493732430739748,
-1.5895375549615));
#58133=CARTESIAN_POINT('Ctrl Pts',(-0.541719566281419,0.0741164881368422,
-1.56592016650372));
#58134=CARTESIAN_POINT('Ctrl Pts',(-0.359721314085519,-0.411988667468349,
-1.54230277804595));
#58135=CARTESIAN_POINT('Ctrl Pts',(0.146797554499674,-0.526884431740369,
-1.51868538958817));
#58136=CARTESIAN_POINT('Ctrl Pts',(0.520854846090516,-0.166749044115146,
-1.49506800113039));
#58137=CARTESIAN_POINT('Ctrl Pts',(0.425472627420327,0.34365269995153,-1.47145061267261));
#58138=CARTESIAN_POINT('Ctrl Pts',(-0.0534762493861652,0.544301818851712,
-1.44783322421483));
#58139=CARTESIAN_POINT('Ctrl Pts',(-0.484201512798375,0.25429349187498,
-1.42421583575705));
#58140=CARTESIAN_POINT('Ctrl Pts',(-0.47846700689053,-0.264934151074547,
-1.40059844729927));
#58141=CARTESIAN_POINT('Ctrl Pts',(-0.0414269475550245,-0.5453477373904,
-1.3769810588415));
#58142=CARTESIAN_POINT('Ctrl Pts',(0.432953585909302,-0.334171471377069,
-1.35336367038372));
#58143=CARTESIAN_POINT('Ctrl Pts',(0.517061852903206,0.178233244978392,
-1.32974628192594));
#58144=CARTESIAN_POINT('Ctrl Pts',(0.13507875124224,0.529975149628081,-1.30612889346816));
#58145=CARTESIAN_POINT('Ctrl Pts',(-0.368666860709707,0.40398584419447,
-1.28251150501038));
#58146=CARTESIAN_POINT('Ctrl Pts',(-0.540088448786064,-0.0861648450742474,
-1.25889411655261));
#58147=CARTESIAN_POINT('Ctrl Pts',(-0.224662619646612,-0.49864475876141,
-1.23527672809483));
#58148=CARTESIAN_POINT('Ctrl Pts',(0.293278862692737,-0.461635554257514,
-1.21165933963705));
#58149=CARTESIAN_POINT('Ctrl Pts',(0.546852512846713,-0.00849817358128052,
-1.18804195117927));
#58150=CARTESIAN_POINT('Ctrl Pts',(0.3074815602605,0.452299652167739,-1.16442456272149));
#58151=CARTESIAN_POINT('Ctrl Pts',(-0.209059860785428,0.505384862046751,
-1.14080717426371));
#58152=CARTESIAN_POINT('Ctrl Pts',(-0.537150241500616,0.102905316020012,
-1.11718978580594));
#58153=CARTESIAN_POINT('Ctrl Pts',(-0.381041867255769,-0.392335291111666,
-1.09357239734816));
#58154=CARTESIAN_POINT('Ctrl Pts',(0.118545820857808,-0.533916448095865,
-1.06995500889038));
#58155=CARTESIAN_POINT('Ctrl Pts',(0.511273763030655,-0.194213863220489,
-1.0463376204326));
#58156=CARTESIAN_POINT('Ctrl Pts',(0.443128564866245,0.320557265258415,
-1.02272023197482));
#58157=CARTESIAN_POINT('Ctrl Pts',(-0.0244622294377454,0.546371196756361,
-0.999102843517045));
#58158=CARTESIAN_POINT('Ctrl Pts',(-0.470002245332516,0.279674408423102,
-0.975485455059269));
#58159=CARTESIAN_POINT('Ctrl Pts',(-0.49187215271962,-0.239126892475631,
-0.951868066601488));
#58160=CARTESIAN_POINT('Ctrl Pts',(-0.0703579478920888,-0.542374081697089,
-0.928250678143711));
#58161=CARTESIAN_POINT('Ctrl Pts',(0.41457842079967,-0.356713636323652,
-0.904633289685933));
#58162=CARTESIAN_POINT('Ctrl Pts',(0.525804905643713,0.150496134602677,
-0.881015901228154));
#58163=CARTESIAN_POINT('Ctrl Pts',(0.163059566697128,0.522045460700883,
-0.857398512770376));
#58164=CARTESIAN_POINT('Ctrl Pts',(-0.346671164332164,0.423011807341991,
-0.833781124312598));
#58165=CARTESIAN_POINT('Ctrl Pts',(-0.543905069539545,-0.0573337654383577,
-0.810163735854821));
#58166=CARTESIAN_POINT('Ctrl Pts',(-0.250851274854172,-0.485997451880037,
-0.786546347397042));
#58167=CARTESIAN_POINT('Ctrl Pts',(0.268325241332186,-0.476572607472738,
-0.762928958939263));
#58168=CARTESIAN_POINT('Ctrl Pts',(0.545627627708702,-0.0375549891887017,
-0.739311570481486));
#58169=CARTESIAN_POINT('Ctrl Pts',(0.331089563293141,0.435315502143794,
-0.715694182023707));
#58170=CARTESIAN_POINT('Ctrl Pts',(-0.181899737431087,0.515783259566058,
-0.692076793565929));
#58171=CARTESIAN_POINT('Ctrl Pts',(-0.530920711956982,0.131312920002222,
-0.66845940510815));
#58172=CARTESIAN_POINT('Ctrl Pts',(-0.4013583650666,-0.371525703155395,
-0.644842016650373));
#58173=CARTESIAN_POINT('Ctrl Pts',(0.0899970236864376,-0.539463085889993,
-0.621224628192594));
#58174=CARTESIAN_POINT('Ctrl Pts',(0.500227164451271,-0.221116868138983,
-0.597607239734816));
#58175=CARTESIAN_POINT('Ctrl Pts',(0.459541805813008,0.296548838979816,
-0.573989851277038));
#58176=CARTESIAN_POINT('Ctrl Pts',(0.00461560395756986,0.546899059656848,
-0.550372462819259));
#58177=CARTESIAN_POINT('Ctrl Pts',(-0.45447120354255,0.304262733767933,
-0.526755074361482));
#58178=CARTESIAN_POINT('Ctrl Pts',(-0.503887914568089,-0.212642549199021,
-0.503137685903703));
#58179=CARTESIAN_POINT('Ctrl Pts',(-0.0990892522675508,-0.537867274833063,
-0.479520297445925));
#58180=CARTESIAN_POINT('Ctrl Pts',(0.395030596686354,-0.378246900109711,
-0.455902908988147));
#58181=CARTESIAN_POINT('Ctrl Pts',(0.53306137339736,0.122333349699535,-0.432285520530368));
#58182=CARTESIAN_POINT('Ctrl Pts',(0.190579222289824,0.512639686464196,
-0.408668132072591));
#58183=CARTESIAN_POINT('Ctrl Pts',(-0.323695189913716,0.440841623562851,
-0.385050743614812));
#58184=CARTESIAN_POINT('Ctrl Pts',(-0.546183695283555,-0.0283405628290827,
-0.361433355157034));
#58185=CARTESIAN_POINT('Ctrl Pts',(-0.276330724342253,-0.471975909390466,
-0.337815966699255));
#58186=CARTESIAN_POINT('Ctrl Pts',(0.24261312478672,-0.490162137485593,
-0.314198578241477));
#58187=CARTESIAN_POINT('Ctrl Pts',(0.542859462318489,-0.0665055186080004,
-0.290581189783699));
#58188=CARTESIAN_POINT('Ctrl Pts',(0.353762239687556,0.417100257050748,
-0.266963801325921));
#58189=CARTESIAN_POINT('Ctrl Pts',(-0.154226947575804,0.524723574589349,
-0.243346412868143));
#58190=CARTESIAN_POINT('Ctrl Pts',(-0.523186708236817,0.159348527858055,
-0.219729024410364));
#58191=CARTESIAN_POINT('Ctrl Pts',(-0.420546184709156,-0.34966424721476,
-0.196111635952586));
#58192=CARTESIAN_POINT('Ctrl Pts',(0.0612057012012895,-0.543486887614036,
-0.172494247494808));
#58193=CARTESIAN_POINT('Ctrl Pts',(0.487743116733933,-0.247389705703288,
-0.14887685903703));
#58194=CARTESIAN_POINT('Ctrl Pts',(0.47469987174551,0.271692396254022,-0.125259470579251));
#58195=CARTESIAN_POINT('Ctrl Pts',(0.0335952617984759,0.545898749141681,
-0.101642082121473));
#58196=CARTESIAN_POINT('Ctrl Pts',(-0.437491108098618,0.327955595531638,
-0.0780246936636949));
#58197=CARTESIAN_POINT('Ctrl Pts',(-0.514796402181575,-0.185489273660303,
-0.0544073052059169));
#58198=CARTESIAN_POINT('Ctrl Pts',(-0.126910101031704,-0.531970590082557,
-0.0307899167481385));
#58199=CARTESIAN_POINT('Ctrl Pts',(0.289659225408945,-0.420705977806036,
-0.0111087596999904));
#58200=CARTESIAN_POINT('Ctrl Pts',(0.457939177385175,-0.15232207079224,
0.0046361659385287));
#58201=CARTESIAN_POINT('Ctrl Pts',(0.470262631272262,0.00422963406109354,
0.012508628757788));
#58202=CARTESIAN_POINT('Ctrl Pts',(0.457137697731917,0.0796027151346424,
0.0164448601674178));
#58203=CARTESIAN_POINT('Ctrl Pts',(0.252761008811552,-0.354684587865065,
-1.64394486016742));
#58204=CARTESIAN_POINT('Ctrl Pts',(0.311241572390819,-0.313009232487664,
-1.64000862875779));
#58205=CARTESIAN_POINT('Ctrl Pts',(0.406273582278792,-0.200338778311071,
-1.63213616593853));
#58206=CARTESIAN_POINT('Ctrl Pts',(0.470925553959198,0.0898796080548794,
-1.61639124030001));
#58207=CARTESIAN_POINT('Ctrl Pts',(0.266139401546332,0.43894848281088,-1.59671008325186));
#58208=CARTESIAN_POINT('Ctrl Pts',(-0.221421601042844,0.463425016346075,
-1.57309269479408));
#58209=CARTESIAN_POINT('Ctrl Pts',(-0.508466495674223,0.0695669001828929,
-1.54947530633631));
#58210=CARTESIAN_POINT('Ctrl Pts',(-0.337640076853661,-0.386699035892494,
-1.52585791787853));
#58211=CARTESIAN_POINT('Ctrl Pts',(0.137786490937306,-0.494542005324496,
-1.50224052942075));
#58212=CARTESIAN_POINT('Ctrl Pts',(0.48888254150488,-0.156513272541107,
-1.47862314096297));
#58213=CARTESIAN_POINT('Ctrl Pts',(0.399355292545094,0.322557823179248,
-1.45500575250519));
#58214=CARTESIAN_POINT('Ctrl Pts',(-0.0501936478200969,0.510890238505547,
-1.43138836404742));
#58215=CARTESIAN_POINT('Ctrl Pts',(-0.454479147029459,0.238683866588015,
-1.40777097558963));
#58216=CARTESIAN_POINT('Ctrl Pts',(-0.449096649691581,-0.248671356484325,
-1.38415358713186));
#58217=CARTESIAN_POINT('Ctrl Pts',(-0.0388839838191108,-0.511871954078012,
-1.36053619867408));
#58218=CARTESIAN_POINT('Ctrl Pts',(0.406377037713513,-0.313658593083062,
-1.3369188102163));
#58219=CARTESIAN_POINT('Ctrl Pts',(0.48532237850891,0.167292523895527,-1.31330142175852));
#58220=CARTESIAN_POINT('Ctrl Pts',(0.126787038089945,0.497443001691069,
-1.28968403330074));
#58221=CARTESIAN_POINT('Ctrl Pts',(-0.34603650745541,0.379187460238132,
-1.26606664484297));
#58222=CARTESIAN_POINT('Ctrl Pts',(-0.506935503167179,-0.0808756772917736,
-1.24244925638519));
#58223=CARTESIAN_POINT('Ctrl Pts',(-0.210871864394426,-0.468035804603038,
-1.21883186792741));
#58224=CARTESIAN_POINT('Ctrl Pts',(0.275276148122791,-0.433298383817296,
-1.19521447946963));
#58225=CARTESIAN_POINT('Ctrl Pts',(0.513284359962297,-0.00797651923515602,
-1.17159709101185));
#58226=CARTESIAN_POINT('Ctrl Pts',(0.288607023193397,0.424535559442814,
-1.14797970255408));
#58227=CARTESIAN_POINT('Ctrl Pts',(-0.196226869797954,0.474362171438012,
-1.1243623140963));
#58228=CARTESIAN_POINT('Ctrl Pts',(-0.504177655647933,0.0965885463250207,
-1.10074492563852));
#58229=CARTESIAN_POINT('Ctrl Pts',(-0.357651883018847,-0.36825206807694,
-1.07712753718074));
#58230=CARTESIAN_POINT('Ctrl Pts',(0.111268969888161,-0.501142366353261,
-1.05351014872296));
#58231=CARTESIAN_POINT('Ctrl Pts',(0.479889586419924,-0.182292183243338,
-1.02989276026518));
#58232=CARTESIAN_POINT('Ctrl Pts',(0.415927432817955,0.30088008533217,-1.00627537180741));
#58233=CARTESIAN_POINT('Ctrl Pts',(-0.0229606328676126,0.512832589118107,
-0.982657983349627));
#58234=CARTESIAN_POINT('Ctrl Pts',(-0.441151491506388,0.262506793610591,
-0.95904059489185));
#58235=CARTESIAN_POINT('Ctrl Pts',(-0.46167893017022,-0.224448258114767,
-0.935423206434071));
#58236=CARTESIAN_POINT('Ctrl Pts',(-0.0660390752600854,-0.509080834126229,
-0.911805817976294));
#58237=CARTESIAN_POINT('Ctrl Pts',(0.389129819055961,-0.334817023253821,
-0.888188429518514));
#58238=CARTESIAN_POINT('Ctrl Pts',(0.493528745170126,0.141258036329054,
-0.864571041060737));
#58239=CARTESIAN_POINT('Ctrl Pts',(0.153050271072494,0.490000071083492,
-0.840953652602958));
#58240=CARTESIAN_POINT('Ctrl Pts',(-0.325391001268926,0.397045528158503,
-0.81733626414518));
#58241=CARTESIAN_POINT('Ctrl Pts',(-0.51051784336796,-0.0538143729907405,
-0.793718875687403));
#58242=CARTESIAN_POINT('Ctrl Pts',(-0.235452947612843,-0.456164843666864,
-0.770101487229624));
#58243=CARTESIAN_POINT('Ctrl Pts',(0.251854287076352,-0.44731853663581,
-0.746484098771846));
#58244=CARTESIAN_POINT('Ctrl Pts',(0.512134663528028,-0.0352497028655255,
-0.722866710314067));
#58245=CARTESIAN_POINT('Ctrl Pts',(0.310765865736731,0.408593969398428,
-0.699249321856289));
#58246=CARTESIAN_POINT('Ctrl Pts',(-0.170733951314579,0.48412227071514,
-0.675631933398512));
#58247=CARTESIAN_POINT('Ctrl Pts',(-0.498330521348366,0.123252369724435,
-0.652014544940732));
#58248=CARTESIAN_POINT('Ctrl Pts',(-0.376721267049329,-0.348719861889185,
-0.628397156482956));
#58249=CARTESIAN_POINT('Ctrl Pts',(0.0844726203431644,-0.506348527728073,
-0.604779768025176));
#58250=CARTESIAN_POINT('Ctrl Pts',(0.469521075444152,-0.207543766323331,
-0.581162379567398));
#58251=CARTESIAN_POINT('Ctrl Pts',(0.431333158633148,0.278345399239273,
-0.55754499110962));
#58252=CARTESIAN_POINT('Ctrl Pts',(0.00433227838867778,0.51332804952957,
-0.533927602651842));
#58253=CARTESIAN_POINT('Ctrl Pts',(-0.426573811679679,0.28558578207764,
-0.510310214194063));
#58254=CARTESIAN_POINT('Ctrl Pts',(-0.472957113016533,-0.19958963742929,
-0.486692825736286));
#58255=CARTESIAN_POINT('Ctrl Pts',(-0.0930067289341476,-0.504850674398822,
-0.463075437278507));
#58256=CARTESIAN_POINT('Ctrl Pts',(0.370781924234325,-0.355028482944828,
-0.43945804882073));
#58257=CARTESIAN_POINT('Ctrl Pts',(0.50033977980747,0.114824003963517,-0.41584066036295));
#58258=CARTESIAN_POINT('Ctrl Pts',(0.178880652163271,0.48117166361418,-0.392223271905173));
#58259=CARTESIAN_POINT('Ctrl Pts',(-0.303825390712448,0.413780873781272,
-0.368605883447394));
#58260=CARTESIAN_POINT('Ctrl Pts',(-0.512656597289963,-0.0266008975198317,
-0.344988494989616));
#58261=CARTESIAN_POINT('Ctrl Pts',(-0.25936835920088,-0.44300400359871,
-0.321371106531837));
#58262=CARTESIAN_POINT('Ctrl Pts',(0.227720490532905,-0.460073883006124,
-0.29775371807406));
#58263=CARTESIAN_POINT('Ctrl Pts',(0.509536420003117,-0.0624231246098999,
-0.274136329616282));
#58264=CARTESIAN_POINT('Ctrl Pts',(0.332046796002844,0.391496854180891,
-0.250518941158503));
#58265=CARTESIAN_POINT('Ctrl Pts',(-0.1447598359991,0.492513790854095,-0.226901552700725));
#58266=CARTESIAN_POINT('Ctrl Pts',(-0.491071263950452,0.149567031715335,
-0.203284164242946));
#58267=CARTESIAN_POINT('Ctrl Pts',(-0.394731256018808,-0.328200355885785,
-0.179666775785168));
#58268=CARTESIAN_POINT('Ctrl Pts',(0.0574486327284271,-0.510125331242771,
-0.15604938732739));
#58269=CARTESIAN_POINT('Ctrl Pts',(0.457803352124247,-0.232203864424348,
-0.132431998869612));
#58270=CARTESIAN_POINT('Ctrl Pts',(0.445560757460351,0.255014751586155,
-0.108814610411834));
#58271=CARTESIAN_POINT('Ctrl Pts',(0.0315330405271981,0.512389142364513,
-0.0851972219540556));
#58272=CARTESIAN_POINT('Ctrl Pts',(-0.410636027327794,0.307824274359137,
-0.0615798334962771));
#58273=CARTESIAN_POINT('Ctrl Pts',(-0.483195990869901,-0.174103146413242,
-0.0379624450384991));
#58274=CARTESIAN_POINT('Ctrl Pts',(-0.119119814667592,-0.499315953451291,
-0.0143450565807207));
#58275=CARTESIAN_POINT('Ctrl Pts',(0.271878699701397,-0.394881240329992,
0.00533610046742732));
#58276=CARTESIAN_POINT('Ctrl Pts',(0.429828906412464,-0.142971888723207,
0.0210810261059466));
#58277=CARTESIAN_POINT('Ctrl Pts',(0.441395893840263,0.00397000098001296,
0.0289534889252056));
#58278=CARTESIAN_POINT('Ctrl Pts',(0.429076625018155,0.0747163590351825,
0.0328897203348354));
#58279=CARTESIAN_POINT('Ctrl Pts',(0.236230756092322,-0.331488661006753,
-1.6275));
#58280=CARTESIAN_POINT('Ctrl Pts',(0.290886764216325,-0.292538821561541,
-1.62356376859037));
#58281=CARTESIAN_POINT('Ctrl Pts',(0.37970379993858,-0.187236873667965,
-1.61569130577111));
#58282=CARTESIAN_POINT('Ctrl Pts',(0.440127613820048,0.0840015945019269,
-1.59994638013259));
#58283=CARTESIAN_POINT('Ctrl Pts',(0.24873421873435,0.410241802988297,-1.58026522308444));
#58284=CARTESIAN_POINT('Ctrl Pts',(-0.206940906255527,0.433117601952402,
-1.55664783462667));
#58285=CARTESIAN_POINT('Ctrl Pts',(-0.475213425067027,0.0650173122289433,
-1.53303044616889));
#58286=CARTESIAN_POINT('Ctrl Pts',(-0.315558839621802,-0.361409404316639,
-1.50941305771111));
#58287=CARTESIAN_POINT('Ctrl Pts',(0.128775427374938,-0.462199578908625,
-1.48579566925333));
#58288=CARTESIAN_POINT('Ctrl Pts',(0.456910236919244,-0.146277500967067,
-1.46217828079555));
#58289=CARTESIAN_POINT('Ctrl Pts',(0.373237957669861,0.301462946406964,
-1.43856089233778));
#58290=CARTESIAN_POINT('Ctrl Pts',(-0.046911046254029,0.477478658159383,
-1.41494350387999));
#58291=CARTESIAN_POINT('Ctrl Pts',(-0.424756781260542,0.22307424130105,
-1.39132611542222));
#58292=CARTESIAN_POINT('Ctrl Pts',(-0.419726292492632,-0.232408561894103,
-1.36770872696444));
#58293=CARTESIAN_POINT('Ctrl Pts',(-0.0363410200831963,-0.478396170765624,
-1.34409133850666));
#58294=CARTESIAN_POINT('Ctrl Pts',(0.379800489517723,-0.293145714789055,
-1.32047395004888));
#58295=CARTESIAN_POINT('Ctrl Pts',(0.453582904114614,0.156351802812663,
-1.2968565615911));
#58296=CARTESIAN_POINT('Ctrl Pts',(0.118495324937651,0.464910853754055,
-1.27323917313333));
#58297=CARTESIAN_POINT('Ctrl Pts',(-0.323406154201114,0.354389076281796,
-1.24962178467555));
#58298=CARTESIAN_POINT('Ctrl Pts',(-0.473782557548294,-0.0755865095093006,
-1.22600439621777));
#58299=CARTESIAN_POINT('Ctrl Pts',(-0.19708110914224,-0.437426850444666,
-1.20238700775999));
#58300=CARTESIAN_POINT('Ctrl Pts',(0.257273433552846,-0.404961213377078,
-1.17876961930221));
#58301=CARTESIAN_POINT('Ctrl Pts',(0.47971620707788,-0.00745486488903116,
-1.15515223084444));
#58302=CARTESIAN_POINT('Ctrl Pts',(0.269732486126293,0.396771466717889,
-1.13153484238666));
#58303=CARTESIAN_POINT('Ctrl Pts',(-0.183393878810481,0.443339480829272,
-1.10791745392888));
#58304=CARTESIAN_POINT('Ctrl Pts',(-0.47120506979525,0.0902717766300294,
-1.0843000654711));
#58305=CARTESIAN_POINT('Ctrl Pts',(-0.334261898781925,-0.344168845042214,
-1.06068267701332));
#58306=CARTESIAN_POINT('Ctrl Pts',(0.103992118918514,-0.468368284610657,
-1.03706528855554));
#58307=CARTESIAN_POINT('Ctrl Pts',(0.448505409809192,-0.170370503266186,
-1.01344790009777));
#58308=CARTESIAN_POINT('Ctrl Pts',(0.388726300769665,0.281202905405924,
-0.989830511639989));
#58309=CARTESIAN_POINT('Ctrl Pts',(-0.0214590362974804,0.479293981479854,
-0.96621312318221));
#58310=CARTESIAN_POINT('Ctrl Pts',(-0.412300737680259,0.245339178798079,
-0.942595734724431));
#58311=CARTESIAN_POINT('Ctrl Pts',(-0.43148570762082,-0.209769623753902,
-0.918978346266655));
#58312=CARTESIAN_POINT('Ctrl Pts',(-0.0617202026280809,-0.475787586555369,
-0.895360957808874));
#58313=CARTESIAN_POINT('Ctrl Pts',(0.363681217312252,-0.31292041018399,
-0.871743569351098));
#58314=CARTESIAN_POINT('Ctrl Pts',(0.461252584696539,0.132019938055431,
-0.848126180893318));
#58315=CARTESIAN_POINT('Ctrl Pts',(0.14304097544786,0.4579546814661,-0.824508792435541));
#58316=CARTESIAN_POINT('Ctrl Pts',(-0.304110838205687,0.371079248975015,
-0.800891403977763));
#58317=CARTESIAN_POINT('Ctrl Pts',(-0.477130617196376,-0.0502949805431236,
-0.777274015519985));
#58318=CARTESIAN_POINT('Ctrl Pts',(-0.220054620371515,-0.42633223545369,
-0.753656627062206));
#58319=CARTESIAN_POINT('Ctrl Pts',(0.235383332820519,-0.418064465798881,
-0.730039238604428));
#58320=CARTESIAN_POINT('Ctrl Pts',(0.478641699347353,-0.0329444165423497,
-0.70642185014665));
#58321=CARTESIAN_POINT('Ctrl Pts',(0.290442168180321,0.381872436653063,
-0.682804461688872));
#58322=CARTESIAN_POINT('Ctrl Pts',(-0.159568165198072,0.452461281864222,
-0.659187073231093));
#58323=CARTESIAN_POINT('Ctrl Pts',(-0.46574033073975,0.115191819446649,
-0.635569684773316));
#58324=CARTESIAN_POINT('Ctrl Pts',(-0.352084169032058,-0.325914020622976,
-0.611952296315536));
#58325=CARTESIAN_POINT('Ctrl Pts',(0.0789482169998913,-0.473233969566154,
-0.588334907857759));
#58326=CARTESIAN_POINT('Ctrl Pts',(0.438814986437033,-0.193970664507679,
-0.56471751939998));
#58327=CARTESIAN_POINT('Ctrl Pts',(0.40312451145329,0.260141959498729,-0.541100130942203));
#58328=CARTESIAN_POINT('Ctrl Pts',(0.00404895281978514,0.479757039402292,
-0.517482742484423));
#58329=CARTESIAN_POINT('Ctrl Pts',(-0.398676419816808,0.266908830387348,
-0.493865354026646));
#58330=CARTESIAN_POINT('Ctrl Pts',(-0.442026311464977,-0.186536725659559,
-0.470247965568867));
#58331=CARTESIAN_POINT('Ctrl Pts',(-0.0869242056007438,-0.471834073964581,
-0.446630577111089));
#58332=CARTESIAN_POINT('Ctrl Pts',(0.346533251782296,-0.331810065779944,
-0.423013188653311));
#58333=CARTESIAN_POINT('Ctrl Pts',(0.467618186217581,0.1073146582275,-0.399395800195533));
#58334=CARTESIAN_POINT('Ctrl Pts',(0.167182082036718,0.449703640764164,
-0.375778411737755));
#58335=CARTESIAN_POINT('Ctrl Pts',(-0.283955591511179,0.386720123999693,
-0.352161023279976));
#58336=CARTESIAN_POINT('Ctrl Pts',(-0.479129499296371,-0.0248612322105807,
-0.328543634822198));
#58337=CARTESIAN_POINT('Ctrl Pts',(-0.242405994059508,-0.414032097806954,
-0.30492624636442));
#58338=CARTESIAN_POINT('Ctrl Pts',(0.21282785627909,-0.429985628526655,
-0.281308857906642));
#58339=CARTESIAN_POINT('Ctrl Pts',(0.476213377687744,-0.0583407306117992,
-0.257691469448864));
#58340=CARTESIAN_POINT('Ctrl Pts',(0.310331352318132,0.365893451311033,
-0.234074080991085));
#58341=CARTESIAN_POINT('Ctrl Pts',(-0.135292724422396,0.460304007118841,
-0.210456692533307));
#58342=CARTESIAN_POINT('Ctrl Pts',(-0.458955819664086,0.139785535572616,
-0.186839304075529));
#58343=CARTESIAN_POINT('Ctrl Pts',(-0.36891632732846,-0.30673646455681,
-0.163221915617751));
#58344=CARTESIAN_POINT('Ctrl Pts',(0.053691564255565,-0.476763774871506,
-0.139604527159972));
#58345=CARTESIAN_POINT('Ctrl Pts',(0.427863587514561,-0.217018023145409,
-0.115987138702194));
#58346=CARTESIAN_POINT('Ctrl Pts',(0.416421643175193,0.238337106918288,
-0.0923697502444159));
#58347=CARTESIAN_POINT('Ctrl Pts',(0.0294708192559207,0.478879535587345,
-0.0687523617866379));
#58348=CARTESIAN_POINT('Ctrl Pts',(-0.38378094655697,0.287692953186636,
-0.0451349733288593));
#58349=CARTESIAN_POINT('Ctrl Pts',(-0.451595579558226,-0.162717019166182,
-0.0215175848710814));
#58350=CARTESIAN_POINT('Ctrl Pts',(-0.111329528303481,-0.466661316820024,
0.00209980358669715));
#58351=CARTESIAN_POINT('Ctrl Pts',(0.254098173993848,-0.369056502853948,
0.0217809606348451));
#58352=CARTESIAN_POINT('Ctrl Pts',(0.401718635439753,-0.133621706654172,
0.0375258862733644));
#58353=CARTESIAN_POINT('Ctrl Pts',(0.412529156408264,0.00371036789893213,
0.0453983490926234));
#58354=CARTESIAN_POINT('Ctrl Pts',(0.401015552304393,0.0698300029357225,
0.0493345805022531));
#58355=CARTESIAN_POINT('',(0.236230756092323,-0.331488661006752,-1.6275));
#58356=CARTESIAN_POINT('Ctrl Pts',(0.236230756092322,-0.331488661006753,
-1.6275));
#58357=CARTESIAN_POINT('Ctrl Pts',(0.290886764216325,-0.292538821561541,
-1.62356376859037));
#58358=CARTESIAN_POINT('Ctrl Pts',(0.37970379993858,-0.187236873667965,
-1.61569130577111));
#58359=CARTESIAN_POINT('Ctrl Pts',(0.440127613820048,0.0840015945019269,
-1.59994638013259));
#58360=CARTESIAN_POINT('Ctrl Pts',(0.24873421873435,0.410241802988297,-1.58026522308444));
#58361=CARTESIAN_POINT('Ctrl Pts',(-0.206940906255527,0.433117601952402,
-1.55664783462667));
#58362=CARTESIAN_POINT('Ctrl Pts',(-0.398091847258176,0.170836854465825,
-1.53981984923431));
#58363=CARTESIAN_POINT('Ctrl Pts',(-0.407523402849101,0.0186763741788699,
-1.53086432666122));
#58364=CARTESIAN_POINT('Ctrl Pts',(-0.407376298364278,0.00025708744754576,
-1.52978126690739));
#58365=CARTESIAN_POINT('Ctrl Pts',(0.217490523462168,0.442550970777086,
-1.6275));
#58366=CARTESIAN_POINT('Ctrl Pts',(0.229873785936919,0.435229072478121,
-1.6275));
#58367=CARTESIAN_POINT('Ctrl Pts',(0.241888345109027,0.427350072398723,
-1.6275));
#58368=CARTESIAN_POINT('Ctrl Pts',(0.253489436678505,0.418913037947499,
-1.6275));
#58369=CARTESIAN_POINT('Ctrl Pts',(0.26909400111095,0.40756442933387,-1.6275));
#58370=CARTESIAN_POINT('Ctrl Pts',(0.283951058071679,0.395206382965558,
-1.6275));
#58371=CARTESIAN_POINT('Ctrl Pts',(0.29801362485445,0.38193863087979,-1.6275));
#58372=CARTESIAN_POINT('Ctrl Pts',(0.304179723820256,0.37612103913581,-1.6275));
#58373=CARTESIAN_POINT('Ctrl Pts',(0.310192895551237,0.370128419510018,
-1.6275));
#58374=CARTESIAN_POINT('Ctrl Pts',(0.316048301481397,0.363968703364519,
-1.6275));
#58375=CARTESIAN_POINT('Ctrl Pts',(0.321171057221113,0.358579713836594,
-1.6275));
#58376=CARTESIAN_POINT('Ctrl Pts',(0.326166199023329,0.353069987265224,
-1.6275));
#58377=CARTESIAN_POINT('Ctrl Pts',(0.331029922274408,0.347447220488589,
-1.6275));
#58378=CARTESIAN_POINT('Ctrl Pts',(0.347707626437665,0.328166756523267,
-1.6275));
#58379=CARTESIAN_POINT('Ctrl Pts',(0.362849782089381,0.307552414743918,
-1.6275));
#58380=CARTESIAN_POINT('Ctrl Pts',(0.376336339682191,0.285831520294907,
-1.6275));
#58381=CARTESIAN_POINT('Ctrl Pts',(0.380637168863404,0.278904781870704,
-1.6275));
#58382=CARTESIAN_POINT('Ctrl Pts',(0.384769260466003,0.271865370017674,
-1.6275));
#58383=CARTESIAN_POINT('Ctrl Pts',(0.38872763572935,0.264720378190483,-1.6275));
#58384=CARTESIAN_POINT('Ctrl Pts',(0.392044668436885,0.25873302984448,-1.6275));
#58385=CARTESIAN_POINT('Ctrl Pts',(0.39523614201862,0.252677756188667,-1.6275));
#58386=CARTESIAN_POINT('Ctrl Pts',(0.398296493420852,0.246566077761106,
-1.6275));
#58387=CARTESIAN_POINT('Ctrl Pts',(0.409424515402449,0.224342848155274,
-1.6275));
#58388=CARTESIAN_POINT('Ctrl Pts',(0.418838518533126,0.201346395773246,
-1.6275));
#58389=CARTESIAN_POINT('Ctrl Pts',(0.426426057057826,0.177786853885461,
-1.6275));
#58390=CARTESIAN_POINT('Ctrl Pts',(0.43120915988183,0.162935171621331,-1.6275));
#58391=CARTESIAN_POINT('Ctrl Pts',(0.435265495789154,0.147859358365366,
-1.6275));
#58392=CARTESIAN_POINT('Ctrl Pts',(0.438556181607127,0.132611327460787,
-1.6275));
#58393=CARTESIAN_POINT('Ctrl Pts',(0.441238679389305,0.120181453766761,
-1.6275));
#58394=CARTESIAN_POINT('Ctrl Pts',(0.443412244707011,0.10763710396386,-1.6275));
#58395=CARTESIAN_POINT('Ctrl Pts',(0.445051357081788,0.0950072324793357,
-1.6275));
#58396=CARTESIAN_POINT('Ctrl Pts',(0.445788460122358,0.0893276239201484,
-1.6275));
#58397=CARTESIAN_POINT('Ctrl Pts',(0.446416615420648,0.0836362528176917,
-1.6275));
#58398=CARTESIAN_POINT('Ctrl Pts',(0.446933498575069,0.0779430764704747,
-1.6275));
#58399=CARTESIAN_POINT('Ctrl Pts',(0.448780347169872,0.0576010810951417,
-1.6275));
#58400=CARTESIAN_POINT('Ctrl Pts',(0.449212658849586,0.0372069469719805,
-1.6275));
#58401=CARTESIAN_POINT('Ctrl Pts',(0.448151065409431,0.0168795242984948,
-1.6275));
#58402=CARTESIAN_POINT('Ctrl Pts',(0.447138952308652,-0.00250044736930644,
-1.6275));
#58403=CARTESIAN_POINT('Ctrl Pts',(0.444768459778025,-0.0218202753828828,
-1.6275));
#58404=CARTESIAN_POINT('Ctrl Pts',(0.441093000560412,-0.0409472522530066,
-1.6275));
#58405=CARTESIAN_POINT('Ctrl Pts',(0.439301856685364,-0.0502683099605581,
-1.6275));
#58406=CARTESIAN_POINT('Ctrl Pts',(0.437200494232106,-0.059543425004239,
-1.6275));
#58407=CARTESIAN_POINT('Ctrl Pts',(0.434793501026647,-0.0687561428327804,
-1.6275));
#58408=CARTESIAN_POINT('Ctrl Pts',(0.432942862506225,-0.0758394243529009,
-1.6275));
#58409=CARTESIAN_POINT('Ctrl Pts',(0.430910134545771,-0.0828893859763431,
-1.6275));
#58410=CARTESIAN_POINT('Ctrl Pts',(0.42870580678396,-0.089872919404206,
-1.6275));
#58411=CARTESIAN_POINT('Ctrl Pts',(0.421643420461461,-0.112247273988906,
-1.6275));
#58412=CARTESIAN_POINT('Ctrl Pts',(0.412811785079023,-0.133992695543228,
-1.6275));
#58413=CARTESIAN_POINT('Ctrl Pts',(0.402317198650698,-0.154877686132675,
-1.6275));
#58414=CARTESIAN_POINT('Ctrl Pts',(0.396514879481031,-0.166424723463121,
-1.6275));
#58415=CARTESIAN_POINT('Ctrl Pts',(0.390203399917708,-0.177708329366564,
-1.6275));
#58416=CARTESIAN_POINT('Ctrl Pts',(0.383395506236066,-0.188684900928916,
-1.6275));
#58417=CARTESIAN_POINT('Ctrl Pts',(0.376698831746601,-0.199482150445549,
-1.6275));
#58418=CARTESIAN_POINT('Ctrl Pts',(0.369521760837345,-0.2099823271372,-1.6275));
#58419=CARTESIAN_POINT('Ctrl Pts',(0.361881405765658,-0.220153922075274,
-1.6275));
#58420=CARTESIAN_POINT('Ctrl Pts',(0.357855430998159,-0.225513697135685,
-1.6275));
#58421=CARTESIAN_POINT('Ctrl Pts',(0.35369907565792,-0.230783846841213,
-1.6275));
#58422=CARTESIAN_POINT('Ctrl Pts',(0.349429698861994,-0.235942223748248,
-1.6275));
#58423=CARTESIAN_POINT('Ctrl Pts',(0.334930822084277,-0.253460160141096,
-1.6275));
#58424=CARTESIAN_POINT('Ctrl Pts',(0.319098064470797,-0.269738417169507,
-1.6275));
#58425=CARTESIAN_POINT('Ctrl Pts',(0.302054477316776,-0.284621826293324,
-1.6275));
#58426=CARTESIAN_POINT('Ctrl Pts',(0.285433046055008,-0.299136585390496,
-1.6275));
#58427=CARTESIAN_POINT('Ctrl Pts',(0.267659006720295,-0.312325323179623,
-1.6275));
#58428=CARTESIAN_POINT('Ctrl Pts',(0.248825326281718,-0.323999848365032,
-1.6275));
#58429=CARTESIAN_POINT('Ctrl Pts',(0.244678256323088,-0.326570512810337,
-1.6275));
#58430=CARTESIAN_POINT('Ctrl Pts',(0.24047975853273,-0.329067566916157,
-1.6275));
#58431=CARTESIAN_POINT('Ctrl Pts',(0.236230756092326,-0.33148866100675,
-1.6275));
#58432=CARTESIAN_POINT('Ctrl Pts',(0.485198770445679,0.0844890712341024,
3.15686374347968E-17));
#58433=CARTESIAN_POINT('Ctrl Pts',(0.499129368704262,0.00448926714217439,
-0.00393623140962976));
#58434=CARTESIAN_POINT('Ctrl Pts',(0.492589408531074,-0.0785914928595512,
-0.00787246281925949));
#58435=CARTESIAN_POINT('Ctrl Pts',(0.466993216289305,-0.155739180663015,
-0.0118086942288893));
#58436=CARTESIAN_POINT('Ctrl Pts',(0.441397024047537,-0.232886868466477,
-0.0157449256385189));
#58437=CARTESIAN_POINT('Ctrl Pts',(0.396744599737189,-0.304101484071678,
-0.0196811570481487));
#58438=CARTESIAN_POINT('Ctrl Pts',(0.33750030762947,-0.359450861903929,
-0.0236173884577784));
#58439=CARTESIAN_POINT('Ctrl Pts',(0.219011723414032,-0.470149617568429,
-0.0314898512770378));
#58440=CARTESIAN_POINT('Ctrl Pts',(0.0421556680091084,-0.517387422141126,
-0.039362314096297));
#58441=CARTESIAN_POINT('Ctrl Pts',(-0.114888430709592,-0.479714686793065,
-0.0472347769155564));
#58442=CARTESIAN_POINT('Ctrl Pts',(-0.271932529428293,-0.442041951445003,
-0.0551072397348157));
#58443=CARTESIAN_POINT('Ctrl Pts',(-0.40916467146077,-0.319458676176184,
-0.0629797025540751));
#58444=CARTESIAN_POINT('Ctrl Pts',(-0.464105638373042,-0.167339985606525,
-0.0708521653733345));
#58445=CARTESIAN_POINT('Ctrl Pts',(-0.483329384560808,-0.11411392748862,
-0.073606726052103));
#58446=CARTESIAN_POINT('Ctrl Pts',(-0.492478324217231,-0.057271885098475,
-0.0763612867308716));
#58447=CARTESIAN_POINT('Ctrl Pts',(-0.492093596265288,-0.000318355522334279,
-0.0791158474096402));
#58448=CARTESIAN_POINT('Origin',(0.,0.,-1.90478126690739));
#58449=CARTESIAN_POINT('',(-0.236230756092322,-0.331488661006753,-1.6275));
#58450=CARTESIAN_POINT('Ctrl Pts',(-0.236809196450266,-0.331691137924159,
-1.6275));
#58451=CARTESIAN_POINT('Ctrl Pts',(-0.13719578617953,-0.401752132096373,
-1.62032747170964));
#58452=CARTESIAN_POINT('Ctrl Pts',(0.143417983013933,-0.451519069382718,
-1.60528248060002));
#58453=CARTESIAN_POINT('Ctrl Pts',(0.458329322630197,-0.141383602456536,
-1.58236502667114));
#58454=CARTESIAN_POINT('Ctrl Pts',(0.37009909626306,0.305320664636155,-1.55874763821336));
#58455=CARTESIAN_POINT('Ctrl Pts',(-0.0519477178791621,0.476983193860142,
-1.53513024975558));
#58456=CARTESIAN_POINT('Ctrl Pts',(-0.361819606070115,0.263531195926594,
-1.51562061471533));
#58457=CARTESIAN_POINT('Ctrl Pts',(-0.406474643984443,0.0644690927340416,
-1.50398344249434));
#58458=CARTESIAN_POINT('Ctrl Pts',(-0.406409642899809,4.34815695103258E-5,
-1.50021873309261));
#58459=CARTESIAN_POINT('Origin',(0.,0.,-1.6275));
#58460=CARTESIAN_POINT('Ctrl Pts',(-0.179217368492188,0.365473442716068,
-1.67683458050225));
#58461=CARTESIAN_POINT('Ctrl Pts',(-0.239476803591809,0.33592399774102,
-1.67289834909262));
#58462=CARTESIAN_POINT('Ctrl Pts',(-0.344225195791861,0.246456180713373,
-1.66502588627336));
#58463=CARTESIAN_POINT('Ctrl Pts',(-0.447929722889861,-0.0113560346107791,
-1.64928096063485));
#58464=CARTESIAN_POINT('Ctrl Pts',(-0.312098364353949,-0.364364201240606,
-1.6295998035867));
#58465=CARTESIAN_POINT('Ctrl Pts',(0.133800103086114,-0.460991086763511,
-1.60598241512892));
#58466=CARTESIAN_POINT('Ctrl Pts',(0.458329322630197,-0.141383602456536,
-1.58236502667114));
#58467=CARTESIAN_POINT('Ctrl Pts',(0.37009909626306,0.305320664636155,-1.55874763821336));
#58468=CARTESIAN_POINT('Ctrl Pts',(-0.0519477178791621,0.476983193860142,
-1.53513024975558));
#58469=CARTESIAN_POINT('Ctrl Pts',(-0.427063128313673,0.218588880389641,
-1.51151286129781));
#58470=CARTESIAN_POINT('Ctrl Pts',(-0.417269064836094,-0.236797291451368,
-1.48789547284003));
#58471=CARTESIAN_POINT('Ctrl Pts',(-0.0313114294066901,-0.478754704371251,
-1.46427808438225));
#58472=CARTESIAN_POINT('Ctrl Pts',(0.382856292689895,-0.28913914624985,
-1.44066069592447));
#58473=CARTESIAN_POINT('Ctrl Pts',(0.451916785881922,0.161105773860312,
-1.41704330746669));
#58474=CARTESIAN_POINT('Ctrl Pts',(0.113605814801219,0.466130064220589,
-1.39342591900891));
#58475=CARTESIAN_POINT('Ctrl Pts',(-0.327109807248698,0.350972856030287,
-1.36980853055114));
#58476=CARTESIAN_POINT('Ctrl Pts',(-0.472962705865375,-0.0805578494149952,
-1.34619114209336));
#58477=CARTESIAN_POINT('Ctrl Pts',(-0.192476314157182,-0.439472483121615,
-1.32257375363558));
#58478=CARTESIAN_POINT('Ctrl Pts',(0.26151206617616,-0.402236929927433,
-1.2989563651778));
#58479=CARTESIAN_POINT('Ctrl Pts',(0.479768010181106,-0.00241651336352132,
-1.27533897672002));
#58480=CARTESIAN_POINT('Ctrl Pts',(0.265550697114187,0.399582270810862,
-1.25172158826225));
#58481=CARTESIAN_POINT('Ctrl Pts',(-0.188039671187417,0.44138898578519,
-1.22810419980447));
#58482=CARTESIAN_POINT('Ctrl Pts',(-0.472127066500839,0.0853182174774826,
-1.20448681134669));
#58483=CARTESIAN_POINT('Ctrl Pts',(-0.330628982897472,-0.347660232609956,
-1.18086942288891));
#58484=CARTESIAN_POINT('Ctrl Pts',(0.108905154226429,-0.467250284345138,
-1.15725203443113));
#58485=CARTESIAN_POINT('Ctrl Pts',(0.450269851614892,-0.165650906977965,
-1.13363464597335));
#58486=CARTESIAN_POINT('Ctrl Pts',(0.385751642062305,0.285269753596648,
-1.11001725751558));
#58487=CARTESIAN_POINT('Ctrl Pts',(-0.0264913736532199,0.479042136709866,
-1.0863998690578));
#58488=CARTESIAN_POINT('Ctrl Pts',(-0.414854497170337,0.240995659681838,
-1.06278248060002));
#58489=CARTESIAN_POINT('Ctrl Pts',(-0.429258875462494,-0.214289476063294,
-1.03916509214224));
#58490=CARTESIAN_POINT('Ctrl Pts',(-0.0567200932042535,-0.476409480116128,
-1.01554770368446));
#58491=CARTESIAN_POINT('Ctrl Pts',(0.366947398132722,-0.309083756844029,
-0.991930315226685));
#58492=CARTESIAN_POINT('Ctrl Pts',(0.459840631415877,0.136856696679471,
-0.968312926768907));
#58493=CARTESIAN_POINT('Ctrl Pts',(0.138223653062154,0.459431587358633,
-0.944695538311129));
#58494=CARTESIAN_POINT('Ctrl Pts',(-0.307991091943065,0.367864987482187,
-0.92107814985335));
#58495=CARTESIAN_POINT('Ctrl Pts',(-0.476576058306532,-0.0553030051489224,
-0.897460761395572));
#58496=CARTESIAN_POINT('Ctrl Pts',(-0.215565140139133,-0.428619682337017,
-0.873843372937795));
#58497=CARTESIAN_POINT('Ctrl Pts',(0.239760820588477,-0.415569381260058,
-0.850225984480015));
#58498=CARTESIAN_POINT('Ctrl Pts',(0.478961233248966,-0.0279159233190857,
-0.826608596022238));
#58499=CARTESIAN_POINT('Ctrl Pts',(0.286415713505782,0.384901546875125,
-0.802991207564458));
#58500=CARTESIAN_POINT('Ctrl Pts',(-0.164311075821679,0.450760504139189,
-0.779373819106682));
#58501=CARTESIAN_POINT('Ctrl Pts',(-0.466924335892738,0.110294271304891,
-0.755756430648903));
#58502=CARTESIAN_POINT('Ctrl Pts',(-0.348641981099809,-0.329593584196537,
-0.732139042191125));
#58503=CARTESIAN_POINT('Ctrl Pts',(0.0839137360252065,-0.472378711028833,
-0.708521653733346));
#58504=CARTESIAN_POINT('Ctrl Pts',(0.440827811035869,-0.189351532231765,
-0.684904265275568));
#58505=CARTESIAN_POINT('Ctrl Pts',(0.400370238591211,0.264361180523987,
-0.66128687681779));
#58506=CARTESIAN_POINT('Ctrl Pts',(-0.000989657323522311,0.479773052904378,
-0.637669488360011));
#58507=CARTESIAN_POINT('Ctrl Pts',(-0.401457455034637,0.262707201281293,
-0.614052099902234));
#58508=CARTESIAN_POINT('Ctrl Pts',(-0.440042888698431,-0.191168558417772,
-0.590434711444455));
#58509=CARTESIAN_POINT('Ctrl Pts',(-0.0819642213078552,-0.472720877576032,
-0.566817322986677));
#58510=CARTESIAN_POINT('Ctrl Pts',(0.349998754832881,-0.328152455226764,
-0.543199934528899));
#58511=CARTESIAN_POINT('Ctrl Pts',(0.466465341731633,0.112219631976251,
-0.51958254607112));
#58512=CARTESIAN_POINT('Ctrl Pts',(0.162450064697528,0.451434533625857,
-0.495965157613343));
#58513=CARTESIAN_POINT('Ctrl Pts',(-0.288001193431347,0.383716663357668,
-0.472347769155564));
#58514=CARTESIAN_POINT('Ctrl Pts',(-0.47884198251775,-0.0298916458432992,
-0.448730380697786));
#58515=CARTESIAN_POINT('Ctrl Pts',(-0.238044360971215,-0.416554973675746,
-0.425112992240007));
#58516=CARTESIAN_POINT('Ctrl Pts',(0.217331606272519,-0.427726730571028,
-0.40149560378223));
#58517=CARTESIAN_POINT('Ctrl Pts',(0.476800102102078,-0.0533363964720061,
-0.377878215324451));
#58518=CARTESIAN_POINT('Ctrl Pts',(0.306470944705725,0.369132435561808,
-0.354260826866673));
#58519=CARTESIAN_POINT('Ctrl Pts',(-0.140118061818574,0.458857512735786,
-0.330643438408895));
#58520=CARTESIAN_POINT('Ctrl Pts',(-0.460400941337906,0.134958307945479,
-0.307026049951117));
#58521=CARTESIAN_POINT('Ctrl Pts',(-0.365669879310811,-0.310594683296022,
-0.283408661493338));
#58522=CARTESIAN_POINT('Ctrl Pts',(0.0586864453268738,-0.476171978247222,
-0.259791273035561));
#58523=CARTESIAN_POINT('Ctrl Pts',(0.430136573097502,-0.212515682316106,
-0.236173884577782));
#58524=CARTESIAN_POINT('Ctrl Pts',(0.413861933598501,0.242703054136536,
-0.212556496120004));
#58525=CARTESIAN_POINT('Ctrl Pts',(0.0245048656306335,0.479151271800793,
-0.188939107662225));
#58526=CARTESIAN_POINT('Ctrl Pts',(-0.386906026396146,0.283668364350701,
-0.165321719204448));
#58527=CARTESIAN_POINT('Ctrl Pts',(-0.449619579691367,-0.167492585435993,
-0.141704330746669));
#58528=CARTESIAN_POINT('Ctrl Pts',(-0.106905499254799,-0.467723490470255,
-0.118086942288891));
#58529=CARTESIAN_POINT('Ctrl Pts',(0.331923550485991,-0.346239581300314,
-0.0944695538311125));
#58530=CARTESIAN_POINT('Ctrl Pts',(0.472036117814807,0.0871616494771883,
-0.0708521653733347));
#58531=CARTESIAN_POINT('Ctrl Pts',(0.18569067875618,0.442363687480316,-0.0472347769155563));
#58532=CARTESIAN_POINT('Ctrl Pts',(-0.190742685458467,0.405446943649056,
-0.0275536198674078));
#58533=CARTESIAN_POINT('Ctrl Pts',(-0.374661374851549,0.197130638471333,
-0.0118086942288892));
#58534=CARTESIAN_POINT('Ctrl Pts',(-0.40764782825114,0.0633823306528579,
-0.00393623140962957));
#58535=CARTESIAN_POINT('Ctrl Pts',(-0.407032914766026,-0.00372944996921217,
2.22044604925031E-16));
#58536=CARTESIAN_POINT('Ctrl Pts',(-0.19175810807181,0.391047455474607,
-1.66038972033484));
#58537=CARTESIAN_POINT('Ctrl Pts',(-0.256234198561238,0.359430287391736,
-1.65645348892521));
#58538=CARTESIAN_POINT('Ctrl Pts',(-0.368312361971621,0.263701957761204,
-1.64858102610595));
#58539=CARTESIAN_POINT('Ctrl Pts',(-0.479273615794859,-0.0121506734000261,
-1.63283610046743));
#58540=CARTESIAN_POINT('Ctrl Pts',(-0.333937454747469,-0.389860594800781,
-1.61315494341928));
#58541=CARTESIAN_POINT('Ctrl Pts',(0.14316276844967,-0.493248948913077,
-1.5895375549615));
#58542=CARTESIAN_POINT('Ctrl Pts',(0.490400927771866,-0.151276923367082,
-1.56592016650372));
#58543=CARTESIAN_POINT('Ctrl Pts',(0.395996789237453,0.326685485332349,
-1.54230277804595));
#58544=CARTESIAN_POINT('Ctrl Pts',(-0.0555827606607796,0.510360104080303,
-1.51868538958816));
#58545=CARTESIAN_POINT('Ctrl Pts',(-0.456946880771931,0.23388464244123,
-1.49506800113039));
#58546=CARTESIAN_POINT('Ctrl Pts',(-0.446467477471926,-0.253367187495685,
-1.47145061267261));
#58547=CARTESIAN_POINT('Ctrl Pts',(-0.0335024474166019,-0.512255576081133,
-1.44783322421483));
#58548=CARTESIAN_POINT('Ctrl Pts',(0.409646670784601,-0.309371664815999,
-1.42421583575705));
#58549=CARTESIAN_POINT('Ctrl Pts',(0.483539673613659,0.17237915417916,-1.40059844729927));
#58550=CARTESIAN_POINT('Ctrl Pts',(0.121555384366601,0.498747526438702,
-1.3769810588415));
#58551=CARTESIAN_POINT('Ctrl Pts',(-0.349999323712195,0.375532189894095,
-1.35336367038372));
#58552=CARTESIAN_POINT('Ctrl Pts',(-0.506058282343447,-0.0861948868244116,
-1.32974628192594));
#58553=CARTESIAN_POINT('Ctrl Pts',(-0.205944848771876,-0.470224580474718,
-1.30612889346816));
#58554=CARTESIAN_POINT('Ctrl Pts',(0.279811379163714,-0.430383468569123,
-1.28251150501038));
#58555=CARTESIAN_POINT('Ctrl Pts',(0.51333978798889,-0.00258560894302878,
-1.25889411655261));
#58556=CARTESIAN_POINT('Ctrl Pts',(0.284132613396715,0.427543049618369,
-1.23527672809483));
#58557=CARTESIAN_POINT('Ctrl Pts',(-0.201197751605845,0.472275190457298,
-1.21165933963705));
#58558=CARTESIAN_POINT('Ctrl Pts',(-0.505164169094702,0.0912883617541506,
-1.18804195117927));
#58559=CARTESIAN_POINT('Ctrl Pts',(-0.353764753759849,-0.371987765571934,
-1.16442456272149));
#58560=CARTESIAN_POINT('Ctrl Pts',(0.116525794957417,-0.499946133992841,
-1.14080717426372));
#58561=CARTESIAN_POINT('Ctrl Pts',(0.481777495082518,-0.177242333093732,
-1.11718978580594));
#58562=CARTESIAN_POINT('Ctrl Pts',(0.412744622297515,0.305231511320786,
-1.09357239734816));
#58563=CARTESIAN_POINT('Ctrl Pts',(-0.0283451081482987,0.512563121504412,
-1.06995500889038));
#58564=CARTESIAN_POINT('Ctrl Pts',(-0.443883950376908,0.257859336641929,
-1.0463376204326));
#58565=CARTESIAN_POINT('Ctrl Pts',(-0.459296275379188,-0.22928438719592,
-1.02272023197482));
#58566=CARTESIAN_POINT('Ctrl Pts',(-0.0606890830616055,-0.509746244703545,
-0.999102843517047));
#58567=CARTESIAN_POINT('Ctrl Pts',(0.39262455095624,-0.330711900006067,
-0.975485455059267));
#58568=CARTESIAN_POINT('Ctrl Pts',(0.492017990425408,0.146433247251684,
-0.95186806660149));
#58569=CARTESIAN_POINT('Ctrl Pts',(0.147895856439432,0.491580323500626,
-0.92825067814371));
#58570=CARTESIAN_POINT('Ctrl Pts',(-0.329542775852931,0.393606348642041,
-0.904633289685933));
#58571=CARTESIAN_POINT('Ctrl Pts',(-0.509924479206744,-0.059172834236236,
-0.881015901228153));
#58572=CARTESIAN_POINT('Ctrl Pts',(-0.230649315895502,-0.458612354699706,
-0.857398512770378));
#58573=CARTESIAN_POINT('Ctrl Pts',(0.256538089653934,-0.44464885849764,
-0.833781124312597));
#58574=CARTESIAN_POINT('Ctrl Pts',(0.512476556821929,-0.0298693407105762,
-0.81016373585482));
#58575=CARTESIAN_POINT('Ctrl Pts',(0.306457659801545,0.411835041679595,
-0.786546347397041));
#58576=CARTESIAN_POINT('Ctrl Pts',(-0.175808747220738,0.482302481028755,
-0.762928958939263));
#58577=CARTESIAN_POINT('Ctrl Pts',(-0.499597377289809,0.118012115536152,
-0.739311570481486));
#58578=CARTESIAN_POINT('Ctrl Pts',(-0.373038211935482,-0.352656903010436,
-0.715694182023706));
#58579=CARTESIAN_POINT('Ctrl Pts',(0.089785601679182,-0.505433422454468,
-0.692076793565929));
#58580=CARTESIAN_POINT('Ctrl Pts',(0.47167474749168,-0.20260141015766,-0.66845940510815));
#58581=CARTESIAN_POINT('Ctrl Pts',(0.428386155462701,0.282859860355108,
-0.644842016650373));
#58582=CARTESIAN_POINT('Ctrl Pts',(-0.0010589086180337,0.513345183576842,
-0.621224628192593));
#58583=CARTESIAN_POINT('Ctrl Pts',(-0.429549449902351,0.281090143875969,
-0.597607239734817));
#58584=CARTESIAN_POINT('Ctrl Pts',(-0.470834900195202,-0.204545582793808,
-0.573989851277037));
#58585=CARTESIAN_POINT('Ctrl Pts',(-0.0876996696235889,-0.505799532113863,
-0.55037246281926));
#58586=CARTESIAN_POINT('Ctrl Pts',(0.374489925942464,-0.351114931007076,
-0.526755074361481));
#58587=CARTESIAN_POINT('Ctrl Pts',(0.499106265001477,0.120072203365817,
-0.503137685903703));
#58588=CARTESIAN_POINT('Ctrl Pts',(0.173817511799362,0.483023675744621,
-0.479520297445925));
#58589=CARTESIAN_POINT('Ctrl Pts',(-0.308154083722225,0.41056724591011,
-0.455902908988146));
#58590=CARTESIAN_POINT('Ctrl Pts',(-0.512348961517989,-0.0319833144649325,
-0.432285520530369));
#58591=CARTESIAN_POINT('Ctrl Pts',(-0.254701520734547,-0.445703417765819,
-0.40866813207259));
#58592=CARTESIAN_POINT('Ctrl Pts',(0.232539390538157,-0.45765691861287,
-0.385050743614812));
#58593=CARTESIAN_POINT('Ctrl Pts',(0.510164200472157,-0.0570686120708559,
-0.361433355157034));
#58594=CARTESIAN_POINT('Ctrl Pts',(0.327916256276871,0.39496248643087,-0.337815966699255));
#58595=CARTESIAN_POINT('Ctrl Pts',(-0.149922826493179,0.490966077992531,
-0.314198578241478));
#58596=CARTESIAN_POINT('Ctrl Pts',(-0.492617508047421,0.14440201872134,
-0.290581189783699));
#58597=CARTESIAN_POINT('Ctrl Pts',(-0.391257637724691,-0.332328553572109,
-0.266963801325921));
#58598=CARTESIAN_POINT('Ctrl Pts',(0.0627930307202971,-0.509492123635771,
-0.243346412868143));
#58599=CARTESIAN_POINT('Ctrl Pts',(0.460235389926868,-0.227386472189515,
-0.219729024410364));
#58600=CARTESIAN_POINT('Ctrl Pts',(0.442821932145767,0.259686206063789,
-0.196111635952586));
#58601=CARTESIAN_POINT('Ctrl Pts',(0.0262195941800665,0.512679893325895,
-0.172494247494808));
#58602=CARTESIAN_POINT('Ctrl Pts',(-0.413979784702292,0.303518064824655,
-0.14887685903703));
#58603=CARTESIAN_POINT('Ctrl Pts',(-0.481081720365837,-0.179212883045216,
-0.125259470579251));
#58604=CARTESIAN_POINT('Ctrl Pts',(-0.114386214082072,-0.500452452727704,
-0.101642082121473));
#58605=CARTESIAN_POINT('Ctrl Pts',(0.35514990874585,-0.370467704153455,
-0.0780246936636948));
#58606=CARTESIAN_POINT('Ctrl Pts',(0.505066856272224,0.0932607879514328,
-0.0544073052059168));
#58607=CARTESIAN_POINT('Ctrl Pts',(0.198684388373932,0.473318096926487,
-0.0307899167481386));
#58608=CARTESIAN_POINT('Ctrl Pts',(-0.204089909364149,0.433818103076491,
-0.01110875969999));
#58609=CARTESIAN_POINT('Ctrl Pts',(-0.400878313377581,0.210924859539488,
0.00463616593852857));
#58610=CARTESIAN_POINT('Ctrl Pts',(-0.436172994630421,0.0678175107325275,
0.0125086287577882));
#58611=CARTESIAN_POINT('Ctrl Pts',(-0.43551505255971,-0.00399041831861005,
0.016444860167418));
#58612=CARTESIAN_POINT('Ctrl Pts',(-0.204298847651432,0.416621468233145,
-1.64394486016742));
#58613=CARTESIAN_POINT('Ctrl Pts',(-0.272991593530667,0.382936577042452,
-1.64000862875779));
#58614=CARTESIAN_POINT('Ctrl Pts',(-0.39239952815138,0.280947734809036,
-1.63213616593853));
#58615=CARTESIAN_POINT('Ctrl Pts',(-0.510617508699857,-0.0129453121892735,
-1.61639124030001));
#58616=CARTESIAN_POINT('Ctrl Pts',(-0.355776545140989,-0.415356988360956,
-1.59671008325186));
#58617=CARTESIAN_POINT('Ctrl Pts',(0.152525433813226,-0.525506811062644,
-1.57309269479408));
#58618=CARTESIAN_POINT('Ctrl Pts',(0.522472532913535,-0.161170244277627,
-1.5494753063363));
#58619=CARTESIAN_POINT('Ctrl Pts',(0.421894482211846,0.348050306028543,
-1.52585791787853));
#58620=CARTESIAN_POINT('Ctrl Pts',(-0.0592178034423973,0.543737014300464,
-1.50224052942075));
#58621=CARTESIAN_POINT('Ctrl Pts',(-0.486830633230189,0.249180404492818,
-1.47862314096297));
#58622=CARTESIAN_POINT('Ctrl Pts',(-0.475665890107758,-0.269937083540001,
-1.45500575250519));
#58623=CARTESIAN_POINT('Ctrl Pts',(-0.0356934654265134,-0.545756447791016,
-1.43138836404741));
#58624=CARTESIAN_POINT('Ctrl Pts',(0.436437048879306,-0.329604183382146,
-1.40777097558964));
#58625=CARTESIAN_POINT('Ctrl Pts',(0.515162561345397,0.183652534498008,
-1.38415358713186));
#58626=CARTESIAN_POINT('Ctrl Pts',(0.129504953931983,0.531364988656815,
-1.36053619867408));
#58627=CARTESIAN_POINT('Ctrl Pts',(-0.372888840175693,0.400091523757903,
-1.3369188102163));
#58628=CARTESIAN_POINT('Ctrl Pts',(-0.539153858821517,-0.0918319242338282,
-1.31330142175852));
#58629=CARTESIAN_POINT('Ctrl Pts',(-0.21941338338657,-0.500976677827821,
-1.28968403330075));
#58630=CARTESIAN_POINT('Ctrl Pts',(0.298110692151268,-0.458530007210813,
-1.26606664484297));
#58631=CARTESIAN_POINT('Ctrl Pts',(0.546911565796673,-0.0027547045225358,
-1.24244925638519));
#58632=CARTESIAN_POINT('Ctrl Pts',(0.302714529679244,0.455503828425875,
-1.21883186792741));
#58633=CARTESIAN_POINT('Ctrl Pts',(-0.214355832024272,0.503161395129407,
-1.19521447946963));
#58634=CARTESIAN_POINT('Ctrl Pts',(-0.538201271688565,0.0972585060308188,
-1.17159709101185));
#58635=CARTESIAN_POINT('Ctrl Pts',(-0.376900524622225,-0.396315298533912,
-1.14797970255407));
#58636=CARTESIAN_POINT('Ctrl Pts',(0.124146435688405,-0.532641983640544,
-1.1243623140963));
#58637=CARTESIAN_POINT('Ctrl Pts',(0.513285138550144,-0.1888337592095,-1.10074492563852));
#58638=CARTESIAN_POINT('Ctrl Pts',(0.439737602532723,0.325193269044925,
-1.07712753718074));
#58639=CARTESIAN_POINT('Ctrl Pts',(-0.0301988426433773,0.546084106298956,
-1.05351014872296));
#58640=CARTESIAN_POINT('Ctrl Pts',(-0.472913403583479,0.27472301360202,
-1.02989276026519));
#58641=CARTESIAN_POINT('Ctrl Pts',(-0.489333675295882,-0.244279298328546,
-1.0062753718074));
#58642=CARTESIAN_POINT('Ctrl Pts',(-0.0646580729189583,-0.54308300929096,
-0.982657983349628));
#58643=CARTESIAN_POINT('Ctrl Pts',(0.418301703779759,-0.352340043168106,
-0.959040594891849));
#58644=CARTESIAN_POINT('Ctrl Pts',(0.524195349434937,0.156009797823898,
-0.935423206434071));
#58645=CARTESIAN_POINT('Ctrl Pts',(0.157568059816711,0.523729059642619,
-0.911805817976294));
#58646=CARTESIAN_POINT('Ctrl Pts',(-0.351094459762798,0.419347709801893,
-0.888188429518514));
#58647=CARTESIAN_POINT('Ctrl Pts',(-0.543272900106956,-0.0630426633235498,
-0.864571041060736));
#58648=CARTESIAN_POINT('Ctrl Pts',(-0.245733491651872,-0.488605027062394,
-0.840953652602959));
#58649=CARTESIAN_POINT('Ctrl Pts',(0.273315358719392,-0.473728335735222,
-0.81733626414518));
#58650=CARTESIAN_POINT('Ctrl Pts',(0.545991880394893,-0.031822758102066,
-0.793718875687402));
#58651=CARTESIAN_POINT('Ctrl Pts',(0.326499606097308,0.438768536484064,
-0.770101487229623));
#58652=CARTESIAN_POINT('Ctrl Pts',(-0.187306418619796,0.513844457918322,
-0.746484098771846));
#58653=CARTESIAN_POINT('Ctrl Pts',(-0.53227041868688,0.125729959767414,
-0.722866710314067));
#58654=CARTESIAN_POINT('Ctrl Pts',(-0.397434442771153,-0.375720221824335,
-0.699249321856289));
#58655=CARTESIAN_POINT('Ctrl Pts',(0.0956574673331571,-0.538488133880103,
-0.675631933398511));
#58656=CARTESIAN_POINT('Ctrl Pts',(0.502521683947491,-0.215851288083556,
-0.652014544940732));
#58657=CARTESIAN_POINT('Ctrl Pts',(0.456402072334192,0.301358540186229,
-0.628397156482955));
#58658=CARTESIAN_POINT('Ctrl Pts',(-0.00112815991254549,0.546917314249306,
-0.604779768025176));
#58659=CARTESIAN_POINT('Ctrl Pts',(-0.457641444770064,0.299473086470645,
-0.581162379567398));
#58660=CARTESIAN_POINT('Ctrl Pts',(-0.501626911691973,-0.217922607169844,
-0.55754499110962));
#58661=CARTESIAN_POINT('Ctrl Pts',(-0.0934351179393231,-0.538878186651692,
-0.533927602651841));
#58662=CARTESIAN_POINT('Ctrl Pts',(0.398981097052048,-0.374077406787389,
-0.510310214194063));
#58663=CARTESIAN_POINT('Ctrl Pts',(0.531747188271319,0.127924774755383,
-0.486692825736285));
#58664=CARTESIAN_POINT('Ctrl Pts',(0.185184958901198,0.514612817863385,
-0.463075437278508));
#58665=CARTESIAN_POINT('Ctrl Pts',(-0.328306974013104,0.437417828462551,
-0.439458048820728));
#58666=CARTESIAN_POINT('Ctrl Pts',(-0.545855940518228,-0.0340749830865658,
-0.415840660362951));
#58667=CARTESIAN_POINT('Ctrl Pts',(-0.271358680497878,-0.474851861855891,
-0.392223271905172));
#58668=CARTESIAN_POINT('Ctrl Pts',(0.247747174803796,-0.487587106654712,
-0.368605883447394));
#58669=CARTESIAN_POINT('Ctrl Pts',(0.543528298842236,-0.0608008276697055,
-0.344988494989616));
#58670=CARTESIAN_POINT('Ctrl Pts',(0.349361567848018,0.420792537299932,
-0.321371106531837));
#58671=CARTESIAN_POINT('Ctrl Pts',(-0.159727591167785,0.523074643249275,
-0.29775371807406));
#58672=CARTESIAN_POINT('Ctrl Pts',(-0.524834074756935,0.153845729497202,
-0.274136329616281));
#58673=CARTESIAN_POINT('Ctrl Pts',(-0.416845396138572,-0.354062423848196,
-0.250518941158503));
#58674=CARTESIAN_POINT('Ctrl Pts',(0.0668996161137206,-0.542812269024319,
-0.226901552700725));
#58675=CARTESIAN_POINT('Ctrl Pts',(0.490334206756235,-0.242257262062924,
-0.203284164242946));
#58676=CARTESIAN_POINT('Ctrl Pts',(0.471781930693032,0.276669357991042,
-0.179666775785169));
#58677=CARTESIAN_POINT('Ctrl Pts',(0.0279343227294995,0.546208514850997,
-0.15604938732739));
#58678=CARTESIAN_POINT('Ctrl Pts',(-0.441053543008437,0.323367765298609,
-0.132431998869612));
#58679=CARTESIAN_POINT('Ctrl Pts',(-0.512543861040306,-0.19093318065444,
-0.108814610411833));
#58680=CARTESIAN_POINT('Ctrl Pts',(-0.121866928909346,-0.533181414985152,
-0.0851972219540557));
#58681=CARTESIAN_POINT('Ctrl Pts',(0.378376267005709,-0.394695827006596,
-0.0615798334962771));
#58682=CARTESIAN_POINT('Ctrl Pts',(0.538097594729642,0.0993599264256769,
-0.037962445038499));
#58683=CARTESIAN_POINT('Ctrl Pts',(0.211678097991684,0.504272506372659,
-0.0143450565807208));
#58684=CARTESIAN_POINT('Ctrl Pts',(-0.217437133269832,0.462189262503926,
0.00533610046742779));
#58685=CARTESIAN_POINT('Ctrl Pts',(-0.427095251903613,0.224719080607643,
0.0210810261059464));
#58686=CARTESIAN_POINT('Ctrl Pts',(-0.464698161009703,0.0722526908121974,
0.028953488925206));
#58687=CARTESIAN_POINT('Ctrl Pts',(-0.463997190353394,-0.00425138666800794,
0.0328897203348358));
#58688=CARTESIAN_POINT('Ctrl Pts',(-0.216839587231054,0.442195480991683,
-1.6275));
#58689=CARTESIAN_POINT('Ctrl Pts',(-0.289748988500096,0.406442866693167,
-1.62356376859037));
#58690=CARTESIAN_POINT('Ctrl Pts',(-0.41648669433114,0.298193511856867,
-1.61569130577111));
#58691=CARTESIAN_POINT('Ctrl Pts',(-0.541961401604855,-0.0137399509785201,
-1.59994638013259));
#58692=CARTESIAN_POINT('Ctrl Pts',(-0.377615635534509,-0.440853381921132,
-1.58026522308444));
#58693=CARTESIAN_POINT('Ctrl Pts',(0.161888099176782,-0.55776467321221,
-1.55664783462667));
#58694=CARTESIAN_POINT('Ctrl Pts',(0.554544138055205,-0.171063565188174,
-1.53303044616889));
#58695=CARTESIAN_POINT('Ctrl Pts',(0.447792175186239,0.369415126724738,
-1.50941305771111));
#58696=CARTESIAN_POINT('Ctrl Pts',(-0.0628528462240147,0.577113924520625,
-1.48579566925333));
#58697=CARTESIAN_POINT('Ctrl Pts',(-0.516714385688448,0.264476166544406,
-1.46217828079555));
#58698=CARTESIAN_POINT('Ctrl Pts',(-0.504864302743589,-0.286506979584318,
-1.43856089233777));
#58699=CARTESIAN_POINT('Ctrl Pts',(-0.0378844834364257,-0.579257319500899,
-1.41494350388));
#58700=CARTESIAN_POINT('Ctrl Pts',(0.463227426974013,-0.349836701948294,
-1.39132611542222));
#58701=CARTESIAN_POINT('Ctrl Pts',(0.546785449077134,0.194925914816856,
-1.36770872696444));
#58702=CARTESIAN_POINT('Ctrl Pts',(0.137454523497365,0.563982450874928,
-1.34409133850666));
#58703=CARTESIAN_POINT('Ctrl Pts',(-0.395778356639189,0.424650857621712,
-1.32047395004888));
#58704=CARTESIAN_POINT('Ctrl Pts',(-0.572249435299589,-0.0974689616432452,
-1.2968565615911));
#58705=CARTESIAN_POINT('Ctrl Pts',(-0.232881918001264,-0.531728775180923,
-1.27323917313333));
#58706=CARTESIAN_POINT('Ctrl Pts',(0.316410005138821,-0.486676545852504,
-1.24962178467555));
#58707=CARTESIAN_POINT('Ctrl Pts',(0.580483343604457,-0.00292380010204273,
-1.22600439621777));
#58708=CARTESIAN_POINT('Ctrl Pts',(0.321296445961772,0.483464607233382,
-1.20238700775999));
#58709=CARTESIAN_POINT('Ctrl Pts',(-0.227513912442699,0.534047599801515,
-1.17876961930221));
#58710=CARTESIAN_POINT('Ctrl Pts',(-0.571238374282429,0.103228650307487,
-1.15515223084444));
#58711=CARTESIAN_POINT('Ctrl Pts',(-0.400036295484601,-0.42064283149589,
-1.13153484238666));
#58712=CARTESIAN_POINT('Ctrl Pts',(0.131767076419393,-0.565337833288247,
-1.10791745392888));
#58713=CARTESIAN_POINT('Ctrl Pts',(0.544792782017771,-0.200425185325267,
-1.0843000654711));
#58714=CARTESIAN_POINT('Ctrl Pts',(0.466730582767932,0.345155026769063,
-1.06068267701332));
#58715=CARTESIAN_POINT('Ctrl Pts',(-0.0320525771384556,0.579605091093501,
-1.03706528855555));
#58716=CARTESIAN_POINT('Ctrl Pts',(-0.50194285679005,0.291586690562111,
-1.01344790009777));
#58717=CARTESIAN_POINT('Ctrl Pts',(-0.519371075212576,-0.259274209461172,
-0.989830511639989));
#58718=CARTESIAN_POINT('Ctrl Pts',(-0.0686270627763104,-0.576419773878377,
-0.966213123182209));
#58719=CARTESIAN_POINT('Ctrl Pts',(0.443978856603277,-0.373968186330145,
-0.942595734724432));
#58720=CARTESIAN_POINT('Ctrl Pts',(0.556372708444467,0.165586348396111,
-0.918978346266654));
#58721=CARTESIAN_POINT('Ctrl Pts',(0.167240263193989,0.555877795784612,
-0.895360957808875));
#58722=CARTESIAN_POINT('Ctrl Pts',(-0.372646143672664,0.445089070961746,
-0.871743569351098));
#58723=CARTESIAN_POINT('Ctrl Pts',(-0.576621321007168,-0.0669124924108635,
-0.848126180893318));
#58724=CARTESIAN_POINT('Ctrl Pts',(-0.260817667408242,-0.518597699425083,
-0.824508792435541));
#58725=CARTESIAN_POINT('Ctrl Pts',(0.290092627784849,-0.502807812972804,
-0.800891403977762));
#58726=CARTESIAN_POINT('Ctrl Pts',(0.579507203967856,-0.0337761754935562,
-0.777274015519984));
#58727=CARTESIAN_POINT('Ctrl Pts',(0.346541552393071,0.465702031288534,
-0.753656627062206));
#58728=CARTESIAN_POINT('Ctrl Pts',(-0.198804090018854,0.545386434807889,
-0.730039238604428));
#58729=CARTESIAN_POINT('Ctrl Pts',(-0.564943460083952,0.133447803998676,
-0.706421850146649));
#58730=CARTESIAN_POINT('Ctrl Pts',(-0.421830673606824,-0.398783540638234,
-0.682804461688872));
#58731=CARTESIAN_POINT('Ctrl Pts',(0.101529332987132,-0.571542845305737,
-0.659187073231093));
#58732=CARTESIAN_POINT('Ctrl Pts',(0.533368620403303,-0.229101166009451,
-0.635569684773314));
#58733=CARTESIAN_POINT('Ctrl Pts',(0.484417989205682,0.319857220017349,
-0.611952296315537));
#58734=CARTESIAN_POINT('Ctrl Pts',(-0.00119741120705677,0.58048944492177,
-0.588334907857758));
#58735=CARTESIAN_POINT('Ctrl Pts',(-0.485733439637777,0.317856029065321,
-0.564717519399981));
#58736=CARTESIAN_POINT('Ctrl Pts',(-0.532418923188744,-0.23129963154588,
-0.541100130942202));
#58737=CARTESIAN_POINT('Ctrl Pts',(-0.0991705662550569,-0.571956841189523,
-0.517482742484424));
#58738=CARTESIAN_POINT('Ctrl Pts',(0.423472268161632,-0.397039882567702,
-0.493865354026645));
#58739=CARTESIAN_POINT('Ctrl Pts',(0.564388111541162,0.135777346144949,
-0.470247965568867));
#58740=CARTESIAN_POINT('Ctrl Pts',(0.196552406003033,0.546201959982149,
-0.446630577111089));
#58741=CARTESIAN_POINT('Ctrl Pts',(-0.348459864303983,0.464268411014993,
-0.423013188653311));
#58742=CARTESIAN_POINT('Ctrl Pts',(-0.579362919518467,-0.0361666517081995,
-0.399395800195533));
#58743=CARTESIAN_POINT('Ctrl Pts',(-0.28801584026121,-0.504000305945962,
-0.375778411737754));
#58744=CARTESIAN_POINT('Ctrl Pts',(0.262954959069435,-0.517517294696554,
-0.352161023279976));
#58745=CARTESIAN_POINT('Ctrl Pts',(0.576892397212316,-0.0645330432685549,
-0.328543634822198));
#58746=CARTESIAN_POINT('Ctrl Pts',(0.370806879419165,0.446622588168993,
-0.30492624636442));
#58747=CARTESIAN_POINT('Ctrl Pts',(-0.169532355842391,0.55518320850602,
-0.281308857906642));
#58748=CARTESIAN_POINT('Ctrl Pts',(-0.557050641466449,0.163289440273063,
-0.257691469448863));
#58749=CARTESIAN_POINT('Ctrl Pts',(-0.442433154552453,-0.375796294124282,
-0.234074080991085));
#58750=CARTESIAN_POINT('Ctrl Pts',(0.0710062015071441,-0.576132414412867,
-0.210456692533307));
#58751=CARTESIAN_POINT('Ctrl Pts',(0.520433023585601,-0.257128051936333,
-0.186839304075529));
#58752=CARTESIAN_POINT('Ctrl Pts',(0.500741929240297,0.293652509918295,
-0.163221915617751));
#58753=CARTESIAN_POINT('Ctrl Pts',(0.0296490512789326,0.579737136376098,
-0.139604527159972));
#58754=CARTESIAN_POINT('Ctrl Pts',(-0.468127301314583,0.343217465772564,
-0.115987138702194));
#58755=CARTESIAN_POINT('Ctrl Pts',(-0.544006001714775,-0.202653478263663,
-0.0923697502444158));
#58756=CARTESIAN_POINT('Ctrl Pts',(-0.129347643736619,-0.565910377242601,
-0.0687523617866376));
#58757=CARTESIAN_POINT('Ctrl Pts',(0.401602625265567,-0.418923949859737,
-0.0451349733288594));
#58758=CARTESIAN_POINT('Ctrl Pts',(0.57112833318706,0.105459064899921,-0.0215175848710811));
#58759=CARTESIAN_POINT('Ctrl Pts',(0.224671807609435,0.53522691581883,0.00209980358669695));
#58760=CARTESIAN_POINT('Ctrl Pts',(-0.230784357175514,0.490560421931362,
0.0217809606348456));
#58761=CARTESIAN_POINT('Ctrl Pts',(-0.453312190429645,0.238513301675797,
0.0375258862733641));
#58762=CARTESIAN_POINT('Ctrl Pts',(-0.493223327388984,0.076687870891867,
0.0453983490926238));
#58763=CARTESIAN_POINT('Ctrl Pts',(-0.492479328147078,-0.00451235501740582,
0.0493345805022536));
#58764=CARTESIAN_POINT('Ctrl Pts',(-0.491975623968706,-0.000315807630563663,
-0.100884152590359));
#58765=CARTESIAN_POINT('Ctrl Pts',(-0.492335557319541,-0.0590109204422641,
-0.0980460184750444));
#58766=CARTESIAN_POINT('Ctrl Pts',(-0.48260563446014,-0.117592231258847,
-0.0952078843597301));
#58767=CARTESIAN_POINT('Ctrl Pts',(-0.462249825318384,-0.172217804087446,
-0.0923697502444159));
#58768=CARTESIAN_POINT('Ctrl Pts',(-0.40578654905539,-0.323739111256642,
-0.0844972874251564));
#58769=CARTESIAN_POINT('Ctrl Pts',(-0.267567096396004,-0.444824744249622,
-0.0766248246058969));
#58770=CARTESIAN_POINT('Ctrl Pts',(-0.109965658565945,-0.480869822848968,
-0.0687523617866375));
#58771=CARTESIAN_POINT('Ctrl Pts',(0.0476357792641106,-0.516914901448312,
-0.0608798989673781));
#58772=CARTESIAN_POINT('Ctrl Pts',(0.224619202264837,-0.467919425654025,
-0.0530074361481188));
#58773=CARTESIAN_POINT('Ctrl Pts',(0.341365198418784,-0.356024518630273,
-0.0451349733288595));
#58774=CARTESIAN_POINT('Ctrl Pts',(0.458111194572732,-0.244129611606518,
-0.0372625105096));
#58775=CARTESIAN_POINT('Ctrl Pts',(0.514619763879896,-0.0693352733532978,
-0.0293900476903405));
#58776=CARTESIAN_POINT('Ctrl Pts',(0.48513129427054,0.0896898709264652,
-0.021517584871081));
#58777=CARTESIAN_POINT('Ctrl Pts',(0.458264621493744,0.234576213664697,
-0.0143450565807208));
#58778=CARTESIAN_POINT('Ctrl Pts',(0.360012975466797,0.366372762798936,
-0.00717252829036059));
#58779=CARTESIAN_POINT('Ctrl Pts',(0.230193623813299,0.43607830012599,-3.19189119579733E-16));
#58780=CARTESIAN_POINT('Ctrl Pts',(-0.23680919645027,-0.331691137924157,
-1.6275));
#58781=CARTESIAN_POINT('Ctrl Pts',(-0.247292584852649,-0.325809951452391,
-1.6275));
#58782=CARTESIAN_POINT('Ctrl Pts',(-0.257473874870603,-0.319455449608397,
-1.6275));
#58783=CARTESIAN_POINT('Ctrl Pts',(-0.267315520773458,-0.312635691693424,
-1.6275));
#58784=CARTESIAN_POINT('Ctrl Pts',(-0.283255918048573,-0.301589810592047,
-1.6275));
#58785=CARTESIAN_POINT('Ctrl Pts',(-0.29830631137668,-0.289324966651072,
-1.6275));
#58786=CARTESIAN_POINT('Ctrl Pts',(-0.312429019847057,-0.275993569245607,
-1.6275));
#58787=CARTESIAN_POINT('Ctrl Pts',(-0.319028081099951,-0.269764260735142,
-1.6275));
#58788=CARTESIAN_POINT('Ctrl Pts',(-0.325427356265326,-0.263297962026011,
-1.6275));
#58789=CARTESIAN_POINT('Ctrl Pts',(-0.33160224299967,-0.256630917261684,
-1.6275));
#58790=CARTESIAN_POINT('Ctrl Pts',(-0.343131837484215,-0.244182377579899,
-1.6275));
#58791=CARTESIAN_POINT('Ctrl Pts',(-0.353893273503953,-0.231023434587135,
-1.6275));
#58792=CARTESIAN_POINT('Ctrl Pts',(-0.363862167909662,-0.217252793490027,
-1.6275));
#58793=CARTESIAN_POINT('Ctrl Pts',(-0.369628845525765,-0.209286930422141,
-1.6275));
#58794=CARTESIAN_POINT('Ctrl Pts',(-0.375130174240918,-0.201116096937704,
-1.6275));
#58795=CARTESIAN_POINT('Ctrl Pts',(-0.380360006918044,-0.192757432410251,
-1.6275));
#58796=CARTESIAN_POINT('Ctrl Pts',(-0.383706638921451,-0.187408623769459,
-1.6275));
#58797=CARTESIAN_POINT('Ctrl Pts',(-0.386943361934687,-0.181980584125983,
-1.6275));
#58798=CARTESIAN_POINT('Ctrl Pts',(-0.390064055273672,-0.176485097474883,
-1.6275));
#58799=CARTESIAN_POINT('Ctrl Pts',(-0.401809603024232,-0.155801392329387,
-1.6275));
#58800=CARTESIAN_POINT('Ctrl Pts',(-0.411879168607904,-0.134230471891167,
-1.6275));
#58801=CARTESIAN_POINT('Ctrl Pts',(-0.420209116630589,-0.11202262843158,
-1.6275));
#58802=CARTESIAN_POINT('Ctrl Pts',(-0.428561360146739,-0.0897553446456697,
-1.6275));
#58803=CARTESIAN_POINT('Ctrl Pts',(-0.435165490034037,-0.0668464241376505,
-1.6275));
#58804=CARTESIAN_POINT('Ctrl Pts',(-0.439917512881615,-0.0435147328928931,
-1.6275));
#58805=CARTESIAN_POINT('Ctrl Pts',(-0.441261264724132,-0.0369171208643323,
-1.6275));
#58806=CARTESIAN_POINT('Ctrl Pts',(-0.44245663271589,-0.0302855657760881,
-1.6275));
#58807=CARTESIAN_POINT('Ctrl Pts',(-0.443500544800912,-0.0236247585498435,
-1.6275));
#58808=CARTESIAN_POINT('Ctrl Pts',(-0.444360853499896,-0.0181354549186164,
-1.6275));
#58809=CARTESIAN_POINT('Ctrl Pts',(-0.445117804571293,-0.0126284577914863,
-1.6275));
#58810=CARTESIAN_POINT('Ctrl Pts',(-0.445768845006311,-0.00711771903575371,
-1.6275));
#58811=CARTESIAN_POINT('Ctrl Pts',(-0.448273775275097,0.0140852901325413,
-1.6275));
#58812=CARTESIAN_POINT('Ctrl Pts',(-0.44922037217288,0.035388346232463,
-1.6275));
#58813=CARTESIAN_POINT('Ctrl Pts',(-0.448549344096801,0.0566336200698592,
-1.6275));
#58814=CARTESIAN_POINT('Ctrl Pts',(-0.44794779188052,0.0756792338347052,
-1.6275));
#58815=CARTESIAN_POINT('Ctrl Pts',(-0.446046245694261,0.094679020300777,
-1.6275));
#58816=CARTESIAN_POINT('Ctrl Pts',(-0.442917696630645,0.113525745732605,
-1.6275));
#58817=CARTESIAN_POINT('Ctrl Pts',(-0.441365148422807,0.122878467776527,
-1.6275));
#58818=CARTESIAN_POINT('Ctrl Pts',(-0.439510089744425,0.132193541186416,
-1.6275));
#58819=CARTESIAN_POINT('Ctrl Pts',(-0.437359504525979,0.14145786706078,
-1.6275));
#58820=CARTESIAN_POINT('Ctrl Pts',(-0.435441498202038,0.149720285802278,
-1.6275));
#58821=CARTESIAN_POINT('Ctrl Pts',(-0.433286363153054,0.157948297464406,
-1.6275));
#58822=CARTESIAN_POINT('Ctrl Pts',(-0.430908919908843,0.16609904483546,
-1.6275));
#58823=CARTESIAN_POINT('Ctrl Pts',(-0.423966865940568,0.189898951844565,
-1.6275));
#58824=CARTESIAN_POINT('Ctrl Pts',(-0.415126170774039,0.213084008869322,
-1.6275));
#58825=CARTESIAN_POINT('Ctrl Pts',(-0.404550194275197,0.235430491055452,
-1.6275));
#58826=CARTESIAN_POINT('Ctrl Pts',(-0.39825831902693,0.248724892585953,
-1.6275));
#58827=CARTESIAN_POINT('Ctrl Pts',(-0.391351203164621,0.26172264764223,
-1.6275));
#58828=CARTESIAN_POINT('Ctrl Pts',(-0.383854614334943,0.274375771801172,
-1.6275));
#58829=CARTESIAN_POINT('Ctrl Pts',(-0.377157196255011,0.285680014895611,
-1.6275));
#58830=CARTESIAN_POINT('Ctrl Pts',(-0.369989182253541,0.296709222419132,
-1.6275));
#58831=CARTESIAN_POINT('Ctrl Pts',(-0.36236981407022,0.307441177344186,
-1.6275));
#58832=CARTESIAN_POINT('Ctrl Pts',(-0.35769318479098,0.314028255618716,
-1.6275));
#58833=CARTESIAN_POINT('Ctrl Pts',(-0.352843152564941,0.320507068160506,
-1.6275));
#58834=CARTESIAN_POINT('Ctrl Pts',(-0.347843186588654,0.326848425345271,
-1.6275));
#58835=CARTESIAN_POINT('Ctrl Pts',(-0.332035070403259,0.346897544004338,
-1.6275));
#58836=CARTESIAN_POINT('Ctrl Pts',(-0.314704075298522,0.365617528645167,
-1.6275));
#58837=CARTESIAN_POINT('Ctrl Pts',(-0.296024592620659,0.382867713127237,
-1.6275));
#58838=CARTESIAN_POINT('Ctrl Pts',(-0.277379319890049,0.400086305304992,
-1.6275));
#58839=CARTESIAN_POINT('Ctrl Pts',(-0.257389750250661,0.415841552587856,
-1.6275));
#58840=CARTESIAN_POINT('Ctrl Pts',(-0.236186328215152,0.429966383029456,
-1.6275));
#58841=CARTESIAN_POINT('Ctrl Pts',(-0.229845262913795,0.434190534774904,
-1.6275));
#58842=CARTESIAN_POINT('Ctrl Pts',(-0.22339538478044,0.438268623250253,
-1.6275));
#58843=CARTESIAN_POINT('Ctrl Pts',(-0.216839587231054,0.442195480991683,
-1.6275));
#58844=CARTESIAN_POINT('Origin',(-4.52129938221115E-17,0.,-1.6275));
#58845=CARTESIAN_POINT('',(-0.4925,-6.03138548580072E-17,-1.6275));
#58846=CARTESIAN_POINT('Origin',(0.,0.,-1.6275));
#58847=CARTESIAN_POINT('Origin',(0.,0.,-1.6275));
#58848=CARTESIAN_POINT('Origin',(0.42,0.,-1.7));
#58849=CARTESIAN_POINT('',(-0.42,-5.14351655641888E-17,-1.7));
#58850=CARTESIAN_POINT('Origin',(0.,0.,-1.7));
#58851=CARTESIAN_POINT('Origin',(0.,0.,-1.66));
#58852=CARTESIAN_POINT('',(-0.46,-5.63337527607782E-17,-1.66));
#58853=CARTESIAN_POINT('Origin',(0.,0.,-0.785));
#71464=UNCERTAINTY_MEASURE_WITH_UNIT(LENGTH_MEASURE(0.001),#71493,
'DISTANCE_ACCURACY_VALUE',
'Maximum model space distance between geometric entities at asserted c
onnectivities');
#71471=UNCERTAINTY_MEASURE_WITH_UNIT(LENGTH_MEASURE(0.001),#71493,
'DISTANCE_ACCURACY_VALUE',
'Maximum model space distance between geometric entities at asserted c
onnectivities');
#71485=(
GEOMETRIC_REPRESENTATION_CONTEXT(3)
GLOBAL_UNCERTAINTY_ASSIGNED_CONTEXT((#71464))
GLOBAL_UNIT_ASSIGNED_CONTEXT((#71493,#71495,#71496))
REPRESENTATION_CONTEXT('','3D')
);
#71492=(
GEOMETRIC_REPRESENTATION_CONTEXT(3)
GLOBAL_UNCERTAINTY_ASSIGNED_CONTEXT((#71471))
GLOBAL_UNIT_ASSIGNED_CONTEXT((#71493,#71495,#71496))
REPRESENTATION_CONTEXT('','3D')
);
#71493=(
LENGTH_UNIT()
NAMED_UNIT(*)
SI_UNIT(.CENTI.,.METRE.)
);
#71495=(
NAMED_UNIT(*)
PLANE_ANGLE_UNIT()
SI_UNIT($,.RADIAN.)
);
#71496=(
NAMED_UNIT(*)
SI_UNIT($,.STERADIAN.)
SOLID_ANGLE_UNIT()
);
#71510=SHAPE_DEFINITION_REPRESENTATION(#71530,#71615);
#71530=PRODUCT_DEFINITION_SHAPE('',$,#71636);
#71615=SHAPE_REPRESENTATION('',(#30184),#71485);
#71622=PRODUCT_DEFINITION_CONTEXT('part definition',#71684,'design');
#71636=PRODUCT_DEFINITION('2026-10-19-03-23-06-453',
'15_DIN_580_M10_Eye_Bolt',#71656,#71622);
#71656=PRODUCT_DEFINITION_FORMATION('',$,#71699);
#71684=APPLICATION_CONTEXT(
'Core Data for Automotive Mechanical Design Process');
#71685=PRODUCT_CONTEXT('part definition',#71684,'mechanical');
#71699=PRODUCT('2026-10-19-03-23-06-453','15_DIN_580_M10_Eye_Bolt',$,(#71685));
#71888=COLOUR_RGB('Black',0.12,0.14,0.17);
#71889=FILL_AREA_STYLE_COLOUR('',#71888);
#71890=FILL_AREA_STYLE('',(#71889));
#71891=SURFACE_STYLE_FILL_AREA(#71890);
#71892=SURFACE_SIDE_STYLE('',(#71891));
#71893=SURFACE_STYLE_USAGE(.BOTH.,#71892);
#71894=PRESENTATION_STYLE_ASSIGNMENT((#71893));
ENDSEC;
END-ISO-10303-21;
